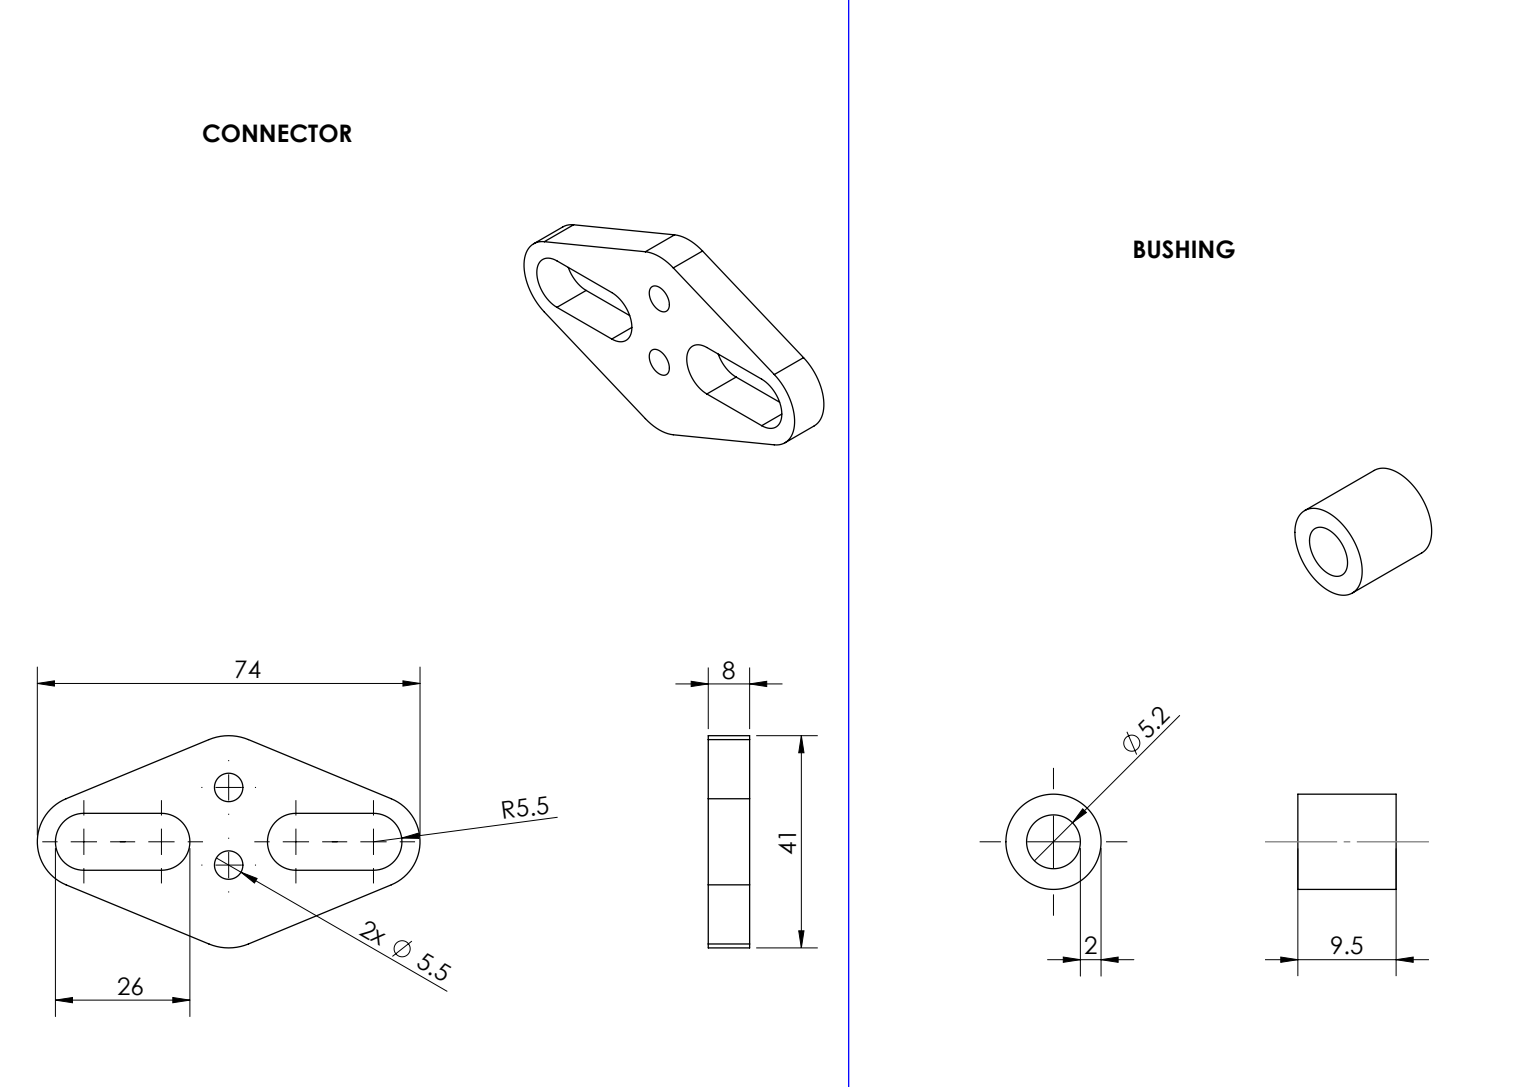
ISO-10303-21;
HEADER;
FILE_DESCRIPTION (('STEP AP214'),
    '1' );
FILE_NAME ('connector.step',
    '2026-09-24T10:26:00',
    ( '' ),
    ( '' ),
    'SwSTEP 2.0',
    'SolidWorks 2026',
    '' );
FILE_SCHEMA (( 'AUTOMOTIVE_DESIGN' ));
ENDSEC;

DATA;
#4=FACE_OUTER_BOUND ( 'NONE', #1590, .T. ) ;
#5=CARTESIAN_POINT ( 'NONE',  ( -13.00000000000000533, 35.49999999999997158, 8.000000000000007105 ) ) ;
#22=CARTESIAN_POINT ( 'NONE',  ( 0.000000000000000000, 25.49999999999996803, 8.000000000000007105 ) ) ;
#36=VERTEX_POINT ( 'NONE', #7746 ) ;
#80=CARTESIAN_POINT ( 'NONE',  ( 2.750000000000003997, 40.49999999999999289, 8.000000000000007105 ) ) ;
#107=EDGE_CURVE ( 'NONE', #8048, #4572, #11469, .T. ) ;
#109=EDGE_CURVE ( 'NONE', #144, #5025, #8095, .T. ) ;
#144=VERTEX_POINT ( 'NONE', #80 ) ;
#167=CARTESIAN_POINT ( 'NONE',  ( 0.000000000000000000, 0.000000000000000000, 0.000000000000000000 ) ) ;
#246=AXIS2_PLACEMENT_3D ( 'NONE', #2195, #9875, #11107 ) ;
#284=VECTOR ( 'NONE', #9089, 1000.000000000000000 ) ;
#288=VECTOR ( 'NONE', #14234, 1000.000000000000000 ) ;
#291=ORIENTED_EDGE ( 'NONE', *, *, #5105, .F. ) ;
#312=EDGE_CURVE ( 'NONE', #10181, #36, #9348, .T. ) ;
#320=ORIENTED_EDGE ( 'NONE', *, *, #6806, .T. ) ;
#341=CARTESIAN_POINT ( 'NONE',  ( 7.500000000000029310, 29.99999999999999289, 0.000000000000000000 ) ) ;
#359=EDGE_LOOP ( 'NONE', ( #6846, #13028, #8516, #4534 ) ) ;
#381=EDGE_CURVE ( 'NONE', #10071, #10068, #6343, .T. ) ;
#397=DIRECTION ( 'NONE',  ( 0.000000000000000000, 0.000000000000000000, -1.000000000000000000 ) ) ;
#405=DIRECTION ( 'NONE',  ( -1.000000000000000000, 0.000000000000000000, 0.000000000000000000 ) ) ;
#413=DIRECTION ( 'NONE',  ( 0.000000000000000000, 0.000000000000000000, 1.000000000000000000 ) ) ;
#414=CARTESIAN_POINT ( 'NONE',  ( -18.12748877629581656, 43.82334295289051340, 8.000000000000007105 ) ) ;
#427=DIRECTION ( 'NONE',  ( 1.000000000000000000, -2.312964634635743450E-16, -0.000000000000000000 ) ) ;
#438=LINE ( 'NONE', #13839, #5839 ) ;
#445=CARTESIAN_POINT ( 'NONE',  ( 28.00000000000000355, 24.50000000000001421, 8.000000000000007105 ) ) ;
#464=AXIS2_PLACEMENT_3D ( 'NONE', #1456, #12793, #10384 ) ;
#503=AXIS2_PLACEMENT_3D ( 'NONE', #5425, #10035, #883 ) ;
#507=CIRCLE ( 'NONE', #2371, 2.750000000000003997 ) ;
#525=CIRCLE ( 'NONE', #4047, 2.749999999999997780 ) ;
#551=ORIENTED_EDGE ( 'NONE', *, *, #3076, .F. ) ;
#572=ORIENTED_EDGE ( 'NONE', *, *, #5224, .F. ) ;
#600=FACE_BOUND ( 'NONE', #2682, .T. ) ;
#610=CARTESIAN_POINT ( 'NONE',  ( 28.00000000000000355, 29.99999999999999645, 8.000000000000007105 ) ) ;
#616=DIRECTION ( 'NONE',  ( -0.3822382184081045131, -0.9240638205168505426, 0.000000000000000000 ) ) ;
#620=EDGE_CURVE ( 'NONE', #11306, #10601, #10148, .T. ) ;
#628=LINE ( 'NONE', #5290, #3064 ) ;
#633=DIRECTION ( 'NONE',  ( 1.000000000000000000, 2.312964634635743943E-16, 0.000000000000000000 ) ) ;
#683=ORIENTED_EDGE ( 'NONE', *, *, #8121, .T. ) ;
#690=CARTESIAN_POINT ( 'NONE',  ( 0.000000000000000000, 40.49999999999999289, 8.000000000000007105 ) ) ;
#697=CARTESIAN_POINT ( 'NONE',  ( -1.734723475976807094E-14, 35.49999999999996447, 8.000000000000007105 ) ) ;
#699=CARTESIAN_POINT ( 'NONE',  ( -28.00000000000000355, 24.50000000000001421, 0.000000000000000000 ) ) ;
#717=DIRECTION ( 'NONE',  ( 0.000000000000000000, 0.000000000000000000, 1.000000000000000000 ) ) ;
#734=AXIS2_PLACEMENT_3D ( 'NONE', #1571, #11524, #13887 ) ;
#780=VERTEX_POINT ( 'NONE', #341 ) ;
#781=ORIENTED_EDGE ( 'NONE', *, *, #5427, .F. ) ;
#791=ORIENTED_EDGE ( 'NONE', *, *, #5224, .T. ) ;
#817=FACE_OUTER_BOUND ( 'NONE', #5758, .T. ) ;
#845=ORIENTED_EDGE ( 'NONE', *, *, #10025, .T. ) ;
#857=DIRECTION ( 'NONE',  ( -0.9240638205168504316, -0.3822382184081046796, 0.000000000000000000 ) ) ;
#880=AXIS2_PLACEMENT_3D ( 'NONE', #8213, #12758, #633 ) ;
#883=DIRECTION ( 'NONE',  ( 1.000000000000000000, 0.000000000000000000, 0.000000000000000000 ) ) ;
#894=LINE ( 'NONE', #5363, #5186 ) ;
#904=VERTEX_POINT ( 'NONE', #6329 ) ;
#912=ADVANCED_FACE ( 'NONE', ( #10802 ), #5239, .T. ) ;
#915=VECTOR ( 'NONE', #4396, 1000.000000000000000 ) ;
#918=DIRECTION ( 'NONE',  ( -0.9240638205168505426, 0.3822382184081045131, 0.000000000000000000 ) ) ;
#937=VERTEX_POINT ( 'NONE', #8951 ) ;
#967=EDGE_CURVE ( 'NONE', #12483, #10071, #11085, .T. ) ;
#974=VERTEX_POINT ( 'NONE', #5712 ) ;
#983=LINE ( 'NONE', #4375, #284 ) ;
#1008=LINE ( 'NONE', #8975, #12593 ) ;
#1020=ADVANCED_FACE ( 'NONE', ( #12260 ), #3623, .T. ) ;
#1027=PRESENTATION_STYLE_ASSIGNMENT (( #3166 ) ) ;
#1039=CARTESIAN_POINT ( 'NONE',  ( -28.00000000000000355, 24.50000000000001421, 8.000000000000007105 ) ) ;
#1069=CYLINDRICAL_SURFACE ( 'NONE', #14439, 5.499999999999980460 ) ;
#1098=LINE ( 'NONE', #5, #8563 ) ;
#1105=CARTESIAN_POINT ( 'NONE',  ( -13.00000000000000533, 29.99999999999999289, 8.000000000000007105 ) ) ;
#1144=DIRECTION ( 'NONE',  ( -1.000000000000000000, 0.000000000000000000, 0.000000000000000000 ) ) ;
#1145=ORIENTED_EDGE ( 'NONE', *, *, #1919, .T. ) ;
#1151=DIRECTION ( 'NONE',  ( 1.000000000000000000, 0.000000000000000000, 0.000000000000000000 ) ) ;
#1155=CARTESIAN_POINT ( 'NONE',  ( -3.822382184081044798, 10.25936179483149324, 8.000000000000007105 ) ) ;
#1205=CARTESIAN_POINT ( 'NONE',  ( 2.750000000000003997, 40.49999999999999289, 0.000000000000000000 ) ) ;
#1262=( NAMED_UNIT ( * ) SI_UNIT ( $, .STERADIAN. ) SOLID_ANGLE_UNIT ( ) );
#1279=DIRECTION ( 'NONE',  ( 0.000000000000000000, 0.000000000000000000, -1.000000000000000000 ) ) ;
#1339=CARTESIAN_POINT ( 'NONE',  ( 6.938893903907228378E-15, 24.50000000000002132, 8.000000000000007105 ) ) ;
#1370=ORIENTED_EDGE ( 'NONE', *, *, #11562, .T. ) ;
#1384=STYLED_ITEM ( 'NONE', ( #1027 ), #1904 ) ;
#1386=EDGE_LOOP ( 'NONE', ( #10991, #9939, #6561, #8171 ) ) ;
#1392=( NAMED_UNIT ( * ) PLANE_ANGLE_UNIT ( ) SI_UNIT ( $, .RADIAN. ) );
#1415=EDGE_CURVE ( 'NONE', #10068, #5462, #7017, .T. ) ;
#1438=LINE ( 'NONE', #7875, #11643 ) ;
#1440=CIRCLE ( 'NONE', #3797, 5.499999999999975131 ) ;
#1456=CARTESIAN_POINT ( 'NONE',  ( -28.00000000000000355, 29.99999999999999645, 8.000000000000007105 ) ) ;
#1461=CARTESIAN_POINT ( 'NONE',  ( 13.00000000000000533, 35.49999999999997158, 0.000000000000000000 ) ) ;
#1463=( GEOMETRIC_REPRESENTATION_CONTEXT ( 3 ) GLOBAL_UNCERTAINTY_ASSIGNED_CONTEXT ( ( #12594 ) ) GLOBAL_UNIT_ASSIGNED_CONTEXT ( ( #1937, #9751, #3116 ) ) REPRESENTATION_CONTEXT ( 'NONE', 'WORKASPACE' ) );
#1500=EDGE_CURVE ( 'NONE', #144, #904, #9130, .T. ) ;
#1522=LINE ( 'NONE', #10104, #2529 ) ;
#1537=EDGE_LOOP ( 'NONE', ( #12834, #4232, #7012, #1145 ) ) ;
#1571=CARTESIAN_POINT ( 'NONE',  ( 28.00000000000000355, 29.99999999999999645, 0.000000000000000000 ) ) ;
#1589=CIRCLE ( 'NONE', #11877, 5.499999999999980460 ) ;
#1590=EDGE_LOOP ( 'NONE', ( #13097, #7525, #7860, #7717 ) ) ;
#1593=EDGE_CURVE ( 'NONE', #5280, #11750, #9299, .T. ) ;
#1607=VECTOR ( 'NONE', #8017, 1000.000000000000000 ) ;
#1629=ADVANCED_FACE ( 'NONE', ( #6815 ), #12659, .F. ) ;
#1635=DIRECTION ( 'NONE',  ( -0.9240638205168504316, -0.3822382184081046796, 0.000000000000000000 ) ) ;
#1657=DIRECTION ( 'NONE',  ( 1.000000000000000000, 0.000000000000000000, 0.000000000000000000 ) ) ;
#1674=EDGE_LOOP ( 'NONE', ( #6926, #2420, #5165, #9689 ) ) ;
#1718=EDGE_LOOP ( 'NONE', ( #3786, #2990 ) ) ;
#1720=DIRECTION ( 'NONE',  ( 0.000000000000000000, 0.000000000000000000, 1.000000000000000000 ) ) ;
#1734=ORIENTED_EDGE ( 'NONE', *, *, #1758, .F. ) ;
#1744=CARTESIAN_POINT ( 'NONE',  ( -13.00000000000000533, 35.49999999999997158, 0.000000000000000000 ) ) ;
#1754=ORIENTED_EDGE ( 'NONE', *, *, #3468, .T. ) ;
#1758=EDGE_CURVE ( 'NONE', #10181, #11306, #2144, .T. ) ;
#1788=VERTEX_POINT ( 'NONE', #12898 ) ;
#1802=ORIENTED_EDGE ( 'NONE', *, *, #10042, .T. ) ;
#1808=CARTESIAN_POINT ( 'NONE',  ( 13.00000000000000533, 29.99999999999999289, 0.000000000000000000 ) ) ;
#1828=FACE_OUTER_BOUND ( 'NONE', #10687, .T. ) ;
#1840=VERTEX_POINT ( 'NONE', #14283 ) ;
#1860=FILL_AREA_STYLE_COLOUR ( '', #12668 ) ;
#1865=VERTEX_POINT ( 'NONE', #8711 ) ;
#1880=VECTOR ( 'NONE', #857, 1000.000000000000114 ) ;
#1898=DIRECTION ( 'NONE',  ( -1.000000000000000000, 0.000000000000000000, 0.000000000000000000 ) ) ;
#1904=MANIFOLD_SOLID_BREP ( 'Boss-Extrude1', #11798 ) ;
#1919=EDGE_CURVE ( 'NONE', #1840, #11047, #9738, .T. ) ;
#1920=CIRCLE ( 'NONE', #8926, 9.000000000000005329 ) ;
#1937=( LENGTH_UNIT ( ) NAMED_UNIT ( * ) SI_UNIT ( .MILLI., .METRE. ) );
#1951=DIRECTION ( 'NONE',  ( 0.000000000000000000, 0.000000000000000000, -1.000000000000000000 ) ) ;
#2011=DIRECTION ( 'NONE',  ( 0.000000000000000000, 0.000000000000000000, -1.000000000000000000 ) ) ;
#2038=AXIS2_PLACEMENT_3D ( 'NONE', #3992, #397, #8135 ) ;
#2042=CYLINDRICAL_SURFACE ( 'NONE', #4497, 5.499999999999984013 ) ;
#2062=VECTOR ( 'NONE', #11153, 1000.000000000000000 ) ;
#2101=DIRECTION ( 'NONE',  ( 0.000000000000000000, 0.000000000000000000, -1.000000000000000000 ) ) ;
#2138=ORIENTED_EDGE ( 'NONE', *, *, #2659, .F. ) ;
#2139=EDGE_CURVE ( 'NONE', #5220, #1840, #12145, .T. ) ;
#2144=CIRCLE ( 'NONE', #4024, 9.000000000000001776 ) ;
#2195=CARTESIAN_POINT ( 'NONE',  ( 0.000000000000000000, 40.49999999999999289, 0.000000000000000000 ) ) ;
#2208=( NAMED_UNIT ( * ) PLANE_ANGLE_UNIT ( ) SI_UNIT ( $, .RADIAN. ) );
#2218=DIRECTION ( 'NONE',  ( 1.000000000000000000, 0.000000000000000000, 0.000000000000000000 ) ) ;
#2236=DIRECTION ( 'NONE',  ( 1.000000000000000000, -2.312964634635743450E-16, -0.000000000000000000 ) ) ;
#2249=CARTESIAN_POINT ( 'NONE',  ( 3.065261730689029740, 7.410293710401357536, 8.000000000000007105 ) ) ;
#2265=ORIENTED_EDGE ( 'NONE', *, *, #3430, .T. ) ;
#2267=VERTEX_POINT ( 'NONE', #14409 ) ;
#2289=CIRCLE ( 'NONE', #8370, 5.499999999999976907 ) ;
#2321=LINE ( 'NONE', #5533, #13804 ) ;
#2334=CARTESIAN_POINT ( 'NONE',  ( 2.750000000000003997, 40.49999999999999289, 8.000000000000007105 ) ) ;
#2360=DIRECTION ( 'NONE',  ( -0.3822382184081050127, -0.9240638205168504316, 0.000000000000000000 ) ) ;
#2361=SURFACE_STYLE_USAGE ( .BOTH. , #7982 ) ;
#2371=AXIS2_PLACEMENT_3D ( 'NONE', #11928, #6421, #14269 ) ;
#2400=LINE ( 'NONE', #3434, #11888 ) ;
#2420=ORIENTED_EDGE ( 'NONE', *, *, #8347, .T. ) ;
#2442=DIRECTION ( 'NONE',  ( -1.000000000000000000, 0.000000000000000000, 0.000000000000000000 ) ) ;
#2462=ORIENTED_EDGE ( 'NONE', *, *, #5881, .T. ) ;
#2474=LINE ( 'NONE', #6923, #10329 ) ;
#2493=ORIENTED_EDGE ( 'NONE', *, *, #10301, .F. ) ;
#2496=DIRECTION ( 'NONE',  ( 0.000000000000000000, 0.000000000000000000, -1.000000000000000000 ) ) ;
#2500=AXIS2_PLACEMENT_3D ( 'NONE', #13365, #11609, #5811 ) ;
#2529=VECTOR ( 'NONE', #427, 1000.000000000000000 ) ;
#2566=( GEOMETRIC_REPRESENTATION_CONTEXT ( 3 ) GLOBAL_UNCERTAINTY_ASSIGNED_CONTEXT ( ( #6305 ) ) GLOBAL_UNIT_ASSIGNED_CONTEXT ( ( #10838, #2208, #14357 ) ) REPRESENTATION_CONTEXT ( 'NONE', 'WORKASPACE' ) );
#2587=AXIS2_PLACEMENT_3D ( 'NONE', #7667, #4199, #14427 ) ;
#2592=DIRECTION ( 'NONE',  ( 1.000000000000000000, 0.000000000000000000, 0.000000000000000000 ) ) ;
#2659=EDGE_CURVE ( 'NONE', #12223, #11750, #9069, .T. ) ;
#2672=DIRECTION ( 'NONE',  ( -1.000000000000000000, 0.000000000000000000, 0.000000000000000000 ) ) ;
#2677=CARTESIAN_POINT ( 'NONE',  ( 7.500000000000029310, 29.99999999999999289, 8.000000000000007105 ) ) ;
#2682=EDGE_LOOP ( 'NONE', ( #6005, #6143, #572, #4410, #10204 ) ) ;
#2690=ORIENTED_EDGE ( 'NONE', *, *, #11605, .T. ) ;
#2714=CARTESIAN_POINT ( 'NONE',  ( -3.822382184081044798, 10.25936179483149324, 0.000000000000000000 ) ) ;
#2721=ADVANCED_FACE ( 'NONE', ( #9165 ), #11227, .T. ) ;
#2767=DIRECTION ( 'NONE',  ( 0.000000000000000000, 0.000000000000000000, -1.000000000000000000 ) ) ;
#2778=AXIS2_PLACEMENT_3D ( 'NONE', #3914, #4929, #9316 ) ;
#2799=EDGE_CURVE ( 'NONE', #12483, #8354, #12334, .T. ) ;
#2801=DIRECTION ( 'NONE',  ( 0.000000000000000000, 0.000000000000000000, 1.000000000000000000 ) ) ;
#2811=CARTESIAN_POINT ( 'NONE',  ( 28.00000000000000355, 29.99999999999999645, 0.000000000000000000 ) ) ;
#2835=EDGE_LOOP ( 'NONE', ( #7365, #10921, #3475, #8407 ) ) ;
#2865=CARTESIAN_POINT ( 'NONE',  ( 18.12748877629582367, 43.82334295289049919, 8.000000000000007105 ) ) ;
#2868=SHAPE_DEFINITION_REPRESENTATION ( #11381, #7856 ) ;
#2871=ORIENTED_EDGE ( 'NONE', *, *, #10301, .T. ) ;
#2876=ADVANCED_FACE ( 'NONE', ( #8284 ), #10414, .F. ) ;
#2905=ORIENTED_EDGE ( 'NONE', *, *, #9218, .F. ) ;
#2921=ORIENTED_EDGE ( 'NONE', *, *, #9960, .T. ) ;
#2945=FACE_BOUND ( 'NONE', #7169, .T. ) ;
#2956=ADVANCED_FACE ( 'NONE', ( #6170 ), #14023, .F. ) ;
#2971=LINE ( 'NONE', #6388, #288 ) ;
#2990=ORIENTED_EDGE ( 'NONE', *, *, #1500, .F. ) ;
#3024=AXIS2_PLACEMENT_3D ( 'NONE', #1105, #8786, #8854 ) ;
#3035=CARTESIAN_POINT ( 'NONE',  ( 13.00000000000000533, 29.99999999999999289, 0.000000000000000000 ) ) ;
#3055=CARTESIAN_POINT ( 'NONE',  ( 3.065261730689029740, 7.410293710401357536, 0.000000000000000000 ) ) ;
#3063=CARTESIAN_POINT ( 'NONE',  ( 0.000000000000000000, 25.49999999999996803, 0.000000000000000000 ) ) ;
#3064=VECTOR ( 'NONE', #10854, 1000.000000000000000 ) ;
#3076=EDGE_CURVE ( 'NONE', #1865, #9330, #1098, .T. ) ;
#3103=AXIS2_PLACEMENT_3D ( 'NONE', #14152, #616, #4062 ) ;
#3116=( NAMED_UNIT ( * ) SI_UNIT ( $, .STERADIAN. ) SOLID_ANGLE_UNIT ( ) );
#3160=DIRECTION ( 'NONE',  ( 1.000000000000000000, 0.000000000000000000, 0.000000000000000000 ) ) ;
#3166=SURFACE_STYLE_USAGE ( .BOTH. , #3232 ) ;
#3171=ADVANCED_FACE ( 'NONE', ( #5288 ), #5007, .T. ) ;
#3205=DIRECTION ( 'NONE',  ( -0.9240638205168504316, -0.3822382184081047352, 0.000000000000000000 ) ) ;
#3222=VECTOR ( 'NONE', #5160, 1000.000000000000000 ) ;
#3225=VERTEX_POINT ( 'NONE', #9607 ) ;
#3232=SURFACE_SIDE_STYLE ('',( #11050 ) ) ;
#3254=LINE ( 'NONE', #9693, #13621 ) ;
#3276=AXIS2_PLACEMENT_3D ( 'NONE', #2865, #2360, #3959 ) ;
#3292=CARTESIAN_POINT ( 'NONE',  ( -13.00000000000000533, 29.99999999999999289, 0.000000000000000000 ) ) ;
#3296=EDGE_LOOP ( 'NONE', ( #5557, #14094 ) ) ;
#3315=ORIENTED_EDGE ( 'NONE', *, *, #1758, .T. ) ;
#3322=LINE ( 'NONE', #1039, #12219 ) ;
#3369=FACE_OUTER_BOUND ( 'NONE', #6945, .T. ) ;
#3370=EDGE_CURVE ( 'NONE', #10504, #11904, #6227, .T. ) ;
#3430=EDGE_CURVE ( 'NONE', #3225, #9041, #1920, .T. ) ;
#3434=CARTESIAN_POINT ( 'NONE',  ( -1.734723475976807094E-14, 35.49999999999996447, 0.000000000000000000 ) ) ;
#3468=EDGE_CURVE ( 'NONE', #7396, #1865, #3793, .T. ) ;
#3475=ORIENTED_EDGE ( 'NONE', *, *, #620, .F. ) ;
#3480=ORIENTED_EDGE ( 'NONE', *, *, #7933, .F. ) ;
#3488=DIRECTION ( 'NONE',  ( -1.000000000000000000, 2.312964634635743943E-16, 0.000000000000000000 ) ) ;
#3527=EDGE_LOOP ( 'NONE', ( #7676, #8823, #7369, #8131 ) ) ;
#3557=DIRECTION ( 'NONE',  ( 0.000000000000000000, 0.000000000000000000, -1.000000000000000000 ) ) ;
#3571=EDGE_LOOP ( 'NONE', ( #14354, #5002 ) ) ;
#3623=CYLINDRICAL_SURFACE ( 'NONE', #9197, 9.000000000000001776 ) ;
#3629=APPLICATION_CONTEXT ( 'automotive_design' ) ;
#3671=AXIS2_PLACEMENT_3D ( 'NONE', #14442, #5568, #10111 ) ;
#3681=VECTOR ( 'NONE', #918, 1000.000000000000000 ) ;
#3685=EDGE_CURVE ( 'NONE', #6397, #10504, #983, .T. ) ;
#3693=CARTESIAN_POINT ( 'NONE',  ( -28.00000000000000355, 29.99999999999999645, 8.000000000000007105 ) ) ;
#3696=CARTESIAN_POINT ( 'NONE',  ( -28.00000000000000355, 29.99999999999999645, 0.000000000000000000 ) ) ;
#3731=FACE_BOUND ( 'NONE', #1718, .T. ) ;
#3785=ORIENTED_EDGE ( 'NONE', *, *, #9218, .T. ) ;
#3786=ORIENTED_EDGE ( 'NONE', *, *, #11283, .F. ) ;
#3793=CIRCLE ( 'NONE', #13617, 5.499999999999975131 ) ;
#3797=AXIS2_PLACEMENT_3D ( 'NONE', #3292, #6708, #4399 ) ;
#3811=FACE_BOUND ( 'NONE', #12655, .T. ) ;
#3820=STYLED_ITEM ( 'NONE', ( #6669 ), #13112 ) ;
#3851=PLANE ( 'NONE',  #880 ) ;
#3861=ORIENTED_EDGE ( 'NONE', *, *, #8889, .T. ) ;
#3879=ADVANCED_FACE ( 'NONE', ( #6895 ), #12916, .F. ) ;
#3880=ORIENTED_EDGE ( 'NONE', *, *, #1415, .F. ) ;
#3914=CARTESIAN_POINT ( 'NONE',  ( 13.00000000000000533, 29.99999999999999289, 8.000000000000007105 ) ) ;
#3945=DIRECTION ( 'NONE',  ( 1.000000000000000000, 4.625929269271485914E-16, 0.000000000000000000 ) ) ;
#3955=CARTESIAN_POINT ( 'NONE',  ( 28.00000000000000355, 35.49999999999997868, 0.000000000000000000 ) ) ;
#3959=DIRECTION ( 'NONE',  ( 0.9240638205168503205, -0.3822382184081049572, -0.000000000000000000 ) ) ;
#3963=DIRECTION ( 'NONE',  ( 0.000000000000000000, 0.000000000000000000, 1.000000000000000000 ) ) ;
#3986=CARTESIAN_POINT ( 'NONE',  ( -28.00000000000000355, 29.99999999999999645, 8.000000000000007105 ) ) ;
#3987=EDGE_LOOP ( 'NONE', ( #11996, #8439, #12869, #2493 ) ) ;
#3992=CARTESIAN_POINT ( 'NONE',  ( -28.00000000000000355, 29.99999999999999645, 8.000000000000007105 ) ) ;
#3994=ORIENTED_EDGE ( 'NONE', *, *, #1415, .T. ) ;
#4015=CIRCLE ( 'NONE', #11708, 2.749999999999997780 ) ;
#4024=AXIS2_PLACEMENT_3D ( 'NONE', #610, #2801, #7241 ) ;
#4040=CARTESIAN_POINT ( 'NONE',  ( 31.44014396567294867, 21.68342561534834090, 8.000000000000007105 ) ) ;
#4047=AXIS2_PLACEMENT_3D ( 'NONE', #22, #10114, #7082 ) ;
#4062=DIRECTION ( 'NONE',  ( 0.9240638205168505426, -0.3822382184081045131, -0.000000000000000000 ) ) ;
#4120=PLANE ( 'NONE',  #4507 ) ;
#4121=CARTESIAN_POINT ( 'NONE',  ( -28.00000000000000355, 29.99999999999999645, 8.000000000000007105 ) ) ;
#4156=ORIENTED_EDGE ( 'NONE', *, *, #11847, .T. ) ;
#4188=ORIENTED_EDGE ( 'NONE', *, *, #6813, .F. ) ;
#4199=DIRECTION ( 'NONE',  ( 0.000000000000000000, 0.000000000000000000, -1.000000000000000000 ) ) ;
#4220=EDGE_CURVE ( 'NONE', #10601, #12223, #11489, .T. ) ;
#4232=ORIENTED_EDGE ( 'NONE', *, *, #5600, .F. ) ;
#4233=DIRECTION ( 'NONE',  ( 1.000000000000000000, 0.000000000000000000, 0.000000000000000000 ) ) ;
#4275=CYLINDRICAL_SURFACE ( 'NONE', #2587, 2.749999999999997780 ) ;
#4296=ORIENTED_EDGE ( 'NONE', *, *, #8889, .F. ) ;
#4326=LINE ( 'NONE', #7645, #7461 ) ;
#4375=CARTESIAN_POINT ( 'NONE',  ( -33.49999999999998579, 29.99999999999999645, 8.000000000000007105 ) ) ;
#4389=ORIENTED_EDGE ( 'NONE', *, *, #5881, .F. ) ;
#4396=DIRECTION ( 'NONE',  ( -1.000000000000000000, 4.625929269271485914E-16, 0.000000000000000000 ) ) ;
#4399=DIRECTION ( 'NONE',  ( 1.000000000000000000, 0.000000000000000000, 0.000000000000000000 ) ) ;
#4406=ORIENTED_EDGE ( 'NONE', *, *, #5896, .F. ) ;
#4410=ORIENTED_EDGE ( 'NONE', *, *, #10256, .T. ) ;
#4414=FILL_AREA_STYLE_COLOUR ( '', #8162 ) ;
#4497=AXIS2_PLACEMENT_3D ( 'NONE', #4121, #8558, #13039 ) ;
#4507=AXIS2_PLACEMENT_3D ( 'NONE', #8324, #3963, #7151 ) ;
#4508=CARTESIAN_POINT ( 'NONE',  ( 28.00000000000000355, 24.50000000000001421, 0.000000000000000000 ) ) ;
#4534=ORIENTED_EDGE ( 'NONE', *, *, #4220, .T. ) ;
#4537=DIRECTION ( 'NONE',  ( -0.9240638205168503205, 0.3822382184081049017, 0.000000000000000000 ) ) ;
#4572=VERTEX_POINT ( 'NONE', #7821 ) ;
#4604=LINE ( 'NONE', #7808, #915 ) ;
#4641=FACE_OUTER_BOUND ( 'NONE', #12693, .T. ) ;
#4692=ORIENTED_EDGE ( 'NONE', *, *, #13091, .F. ) ;
#4693=EDGE_CURVE ( 'NONE', #11306, #2267, #438, .T. ) ;
#4708=VECTOR ( 'NONE', #2496, 1000.000000000000000 ) ;
#4725=DIRECTION ( 'NONE',  ( 0.000000000000000000, 0.000000000000000000, -1.000000000000000000 ) ) ;
#4738=CIRCLE ( 'NONE', #13393, 9.999999999999996447 ) ;
#4743=DIRECTION ( 'NONE',  ( 0.000000000000000000, 0.000000000000000000, -1.000000000000000000 ) ) ;
#4752=ORIENTED_EDGE ( 'NONE', *, *, #1593, .T. ) ;
#4771=DIRECTION ( 'NONE',  ( 0.000000000000000000, 0.000000000000000000, -1.000000000000000000 ) ) ;
#4772=CARTESIAN_POINT ( 'NONE',  ( 0.000000000000000000, 40.49999999999999289, 8.000000000000007105 ) ) ;
#4779=ORIENTED_EDGE ( 'NONE', *, *, #6806, .F. ) ;
#4791=ORIENTED_EDGE ( 'NONE', *, *, #6813, .T. ) ;
#4798=EDGE_LOOP ( 'NONE', ( #1802, #12381, #9453, #10952 ) ) ;
#4800=ORIENTED_EDGE ( 'NONE', *, *, #381, .F. ) ;
#4816=DIRECTION ( 'NONE',  ( 0.000000000000000000, 0.000000000000000000, -1.000000000000000000 ) ) ;
#4834=EDGE_CURVE ( 'NONE', #937, #4572, #4015, .T. ) ;
#4843=EDGE_CURVE ( 'NONE', #904, #8755, #6404, .T. ) ;
#4875=DIRECTION ( 'NONE',  ( 0.3822382184081047352, -0.9240638205168505426, -0.000000000000000000 ) ) ;
#4927=AXIS2_PLACEMENT_3D ( 'NONE', #14166, #8365, #6316 ) ;
#4929=DIRECTION ( 'NONE',  ( 0.000000000000000000, 0.000000000000000000, -1.000000000000000000 ) ) ;
#4931=DIRECTION ( 'NONE',  ( 1.000000000000000000, 0.000000000000000000, 0.000000000000000000 ) ) ;
#4947=DIRECTION ( 'NONE',  ( 1.000000000000000000, 0.000000000000000000, 0.000000000000000000 ) ) ;
#4955=AXIS2_PLACEMENT_3D ( 'NONE', #13724, #9243, #2592 ) ;
#4990=PRODUCT_DEFINITION ( 'UNKNOWN', '', #9904, #13349 ) ;
#4996=VERTEX_POINT ( 'NONE', #6754 ) ;
#5002=ORIENTED_EDGE ( 'NONE', *, *, #9870, .F. ) ;
#5007=CYLINDRICAL_SURFACE ( 'NONE', #6448, 9.000000000000001776 ) ;
#5024=CARTESIAN_POINT ( 'NONE',  ( -13.00000000000000533, 29.99999999999999289, 8.000000000000007105 ) ) ;
#5025=VERTEX_POINT ( 'NONE', #1205 ) ;
#5041=LINE ( 'NONE', #6346, #6303 ) ;
#5071=ORIENTED_EDGE ( 'NONE', *, *, #14458, .T. ) ;
#5105=EDGE_CURVE ( 'NONE', #6397, #9797, #1589, .T. ) ;
#5110=DIRECTION ( 'NONE',  ( 0.000000000000000000, 0.000000000000000000, -1.000000000000000000 ) ) ;
#5151=DIRECTION ( 'NONE',  ( -1.000000000000000000, -4.625929269271486900E-16, 0.000000000000000000 ) ) ;
#5152=ORIENTED_EDGE ( 'NONE', *, *, #7917, .T. ) ;
#5153=AXIS2_PLACEMENT_3D ( 'NONE', #12494, #12427, #9042 ) ;
#5160=DIRECTION ( 'NONE',  ( -0.9240638205168505426, 0.3822382184081045131, 0.000000000000000000 ) ) ;
#5165=ORIENTED_EDGE ( 'NONE', *, *, #2799, .T. ) ;
#5186=VECTOR ( 'NONE', #13070, 1000.000000000000000 ) ;
#5220=VERTEX_POINT ( 'NONE', #10641 ) ;
#5224=EDGE_CURVE ( 'NONE', #974, #11904, #628, .T. ) ;
#5239=CYLINDRICAL_SURFACE ( 'NONE', #13893, 10.00000000000000355 ) ;
#5280=VERTEX_POINT ( 'NONE', #10605 ) ;
#5288=FACE_OUTER_BOUND ( 'NONE', #13955, .T. ) ;
#5290=CARTESIAN_POINT ( 'NONE',  ( -6.938893903907228378E-15, 24.50000000000002132, 0.000000000000000000 ) ) ;
#5293=ORIENTED_EDGE ( 'NONE', *, *, #5636, .F. ) ;
#5308=DIRECTION ( 'NONE',  ( 0.000000000000000000, 0.000000000000000000, 1.000000000000000000 ) ) ;
#5326=CYLINDRICAL_SURFACE ( 'NONE', #6984, 9.999999999999996447 ) ;
#5347=ADVANCED_FACE ( 'NONE', ( #3731, #12505, #7002, #3811, #12639 ), #5900, .T. ) ;
#5363=CARTESIAN_POINT ( 'NONE',  ( -28.00000000000000355, 35.49999999999997868, 8.000000000000007105 ) ) ;
#5425=CARTESIAN_POINT ( 'NONE',  ( 0.000000000000000000, 40.49999999999999289, 8.000000000000007105 ) ) ;
#5427=EDGE_CURVE ( 'NONE', #7396, #9797, #5041, .T. ) ;
#5441=DIRECTION ( 'NONE',  ( 1.000000000000000000, 0.000000000000000000, 0.000000000000000000 ) ) ;
#5462=VERTEX_POINT ( 'NONE', #3955 ) ;
#5481=EDGE_CURVE ( 'NONE', #11750, #3225, #6479, .T. ) ;
#5512=ORIENTED_EDGE ( 'NONE', *, *, #967, .F. ) ;
#5533=CARTESIAN_POINT ( 'NONE',  ( -3.822382184081044798, 10.25936179483149324, 8.000000000000007105 ) ) ;
#5557=ORIENTED_EDGE ( 'NONE', *, *, #13465, .T. ) ;
#5568=DIRECTION ( 'NONE',  ( 0.000000000000000000, 0.000000000000000000, 1.000000000000000000 ) ) ;
#5600=EDGE_CURVE ( 'NONE', #11470, #11163, #2321, .T. ) ;
#5615=DIRECTION ( 'NONE',  ( 0.000000000000000000, 0.000000000000000000, -1.000000000000000000 ) ) ;
#5631=CARTESIAN_POINT ( 'NONE',  ( -2.749999999999997780, 25.49999999999996803, 8.000000000000007105 ) ) ;
#5636=EDGE_CURVE ( 'NONE', #2267, #12223, #4326, .T. ) ;
#5712=CARTESIAN_POINT ( 'NONE',  ( -13.00000000000000533, 24.50000000000001421, 0.000000000000000000 ) ) ;
#5716=DIRECTION ( 'NONE',  ( 2.312964634635743943E-16, 1.000000000000000000, 0.000000000000000000 ) ) ;
#5749=CARTESIAN_POINT ( 'NONE',  ( -31.44014396567295577, 21.68342561534834445, 8.000000000000007105 ) ) ;
#5758=EDGE_LOOP ( 'NONE', ( #10144, #11076, #1754, #6948 ) ) ;
#5803=ADVANCED_FACE ( 'NONE', ( #9260 ), #8155, .F. ) ;
#5811=DIRECTION ( 'NONE',  ( 1.000000000000000000, 0.000000000000000000, 0.000000000000000000 ) ) ;
#5839=VECTOR ( 'NONE', #7892, 1000.000000000000000 ) ;
#5869=ORIENTED_EDGE ( 'NONE', *, *, #13068, .T. ) ;
#5881=EDGE_CURVE ( 'NONE', #11189, #780, #8881, .T. ) ;
#5888=LINE ( 'NONE', #13685, #7711 ) ;
#5894=CARTESIAN_POINT ( 'NONE',  ( 13.00000000000000533, 29.99999999999999289, 8.000000000000007105 ) ) ;
#5896=EDGE_CURVE ( 'NONE', #8969, #5220, #8182, .T. ) ;
#5899=ORIENTED_EDGE ( 'NONE', *, *, #9224, .T. ) ;
#5900=PLANE ( 'NONE',  #464 ) ;
#6005=ORIENTED_EDGE ( 'NONE', *, *, #6624, .T. ) ;
#6009=CARTESIAN_POINT ( 'NONE',  ( -28.00000000000000355, 24.50000000000001421, 8.000000000000007105 ) ) ;
#6019=AXIS2_PLACEMENT_3D ( 'NONE', #9392, #12602, #2672 ) ;
#6060=ORIENTED_EDGE ( 'NONE', *, *, #7237, .F. ) ;
#6143=ORIENTED_EDGE ( 'NONE', *, *, #3370, .T. ) ;
#6170=FACE_OUTER_BOUND ( 'NONE', #11038, .T. ) ;
#6173=EDGE_CURVE ( 'NONE', #5280, #8969, #14019, .T. ) ;
#6227=CIRCLE ( 'NONE', #3671, 5.499999999999980460 ) ;
#6242=VECTOR ( 'NONE', #3205, 1000.000000000000000 ) ;
#6294=CIRCLE ( 'NONE', #11666, 5.499999999999980460 ) ;
#6303=VECTOR ( 'NONE', #9721, 1000.000000000000000 ) ;
#6305=UNCERTAINTY_MEASURE_WITH_UNIT (LENGTH_MEASURE( 1.000000000000000082E-05 ), #10838, 'distance_accuracy_value', 'NONE');
#6312=SURFACE_STYLE_FILL_AREA ( #6599 ) ;
#6316=DIRECTION ( 'NONE',  ( -1.000000000000000000, 0.000000000000000000, 0.000000000000000000 ) ) ;
#6329=CARTESIAN_POINT ( 'NONE',  ( -2.750000000000003997, 40.49999999999999289, 8.000000000000007105 ) ) ;
#6343=LINE ( 'NONE', #7726, #13187 ) ;
#6346=CARTESIAN_POINT ( 'NONE',  ( -6.938893903907228378E-15, 24.50000000000002132, 8.000000000000007105 ) ) ;
#6348=CIRCLE ( 'NONE', #4955, 2.749999999999997780 ) ;
#6369=( GEOMETRIC_REPRESENTATION_CONTEXT ( 3 ) GLOBAL_UNCERTAINTY_ASSIGNED_CONTEXT ( ( #10848 ) ) GLOBAL_UNIT_ASSIGNED_CONTEXT ( ( #11208, #1392, #1262 ) ) REPRESENTATION_CONTEXT ( 'NONE', 'WORKASPACE' ) );
#6388=CARTESIAN_POINT ( 'NONE',  ( 1.734723475976807094E-14, 35.49999999999996447, 8.000000000000007105 ) ) ;
#6397=VERTEX_POINT ( 'NONE', #9510 ) ;
#6399=DIRECTION ( 'NONE',  ( -1.000000000000000000, 0.000000000000000000, 0.000000000000000000 ) ) ;
#6404=LINE ( 'NONE', #7144, #7251 ) ;
#6414=ADVANCED_FACE ( 'NONE', ( #8399 ), #10179, .F. ) ;
#6421=DIRECTION ( 'NONE',  ( 0.000000000000000000, 0.000000000000000000, 1.000000000000000000 ) ) ;
#6448=AXIS2_PLACEMENT_3D ( 'NONE', #3986, #8431, #7400 ) ;
#6479=LINE ( 'NONE', #7580, #1880 ) ;
#6484=AXIS2_PLACEMENT_3D ( 'NONE', #3696, #1720, #4931 ) ;
#6524=DIRECTION ( 'NONE',  ( 0.000000000000000000, 0.000000000000000000, 1.000000000000000000 ) ) ;
#6544=ADVANCED_FACE ( 'NONE', ( #1828 ), #5326, .T. ) ;
#6545=DIRECTION ( 'NONE',  ( 0.000000000000000000, 0.000000000000000000, 1.000000000000000000 ) ) ;
#6552=DIRECTION ( 'NONE',  ( 0.000000000000000000, 0.000000000000000000, -1.000000000000000000 ) ) ;
#6556=DIRECTION ( 'NONE',  ( 0.000000000000000000, 0.000000000000000000, -1.000000000000000000 ) ) ;
#6561=ORIENTED_EDGE ( 'NONE', *, *, #967, .T. ) ;
#6588=CARTESIAN_POINT ( 'NONE',  ( 0.000000000000000000, 19.49999999999999645, 0.000000000000000000 ) ) ;
#6589=CARTESIAN_POINT ( 'NONE',  ( 2.749999999999997780, 25.49999999999996803, 8.000000000000007105 ) ) ;
#6599=FILL_AREA_STYLE ('',( #1860 ) ) ;
#6624=EDGE_CURVE ( 'NONE', #1788, #10504, #6294, .T. ) ;
#6631=EDGE_CURVE ( 'NONE', #14193, #937, #1008, .T. ) ;
#6669=PRESENTATION_STYLE_ASSIGNMENT (( #2361 ) ) ;
#6684=CARTESIAN_POINT ( 'NONE',  ( 6.938893903907228378E-15, 24.50000000000002132, 8.000000000000007105 ) ) ;
#6693=CARTESIAN_POINT ( 'NONE',  ( -3.065261730689029740, 7.410293710401353984, 0.000000000000000000 ) ) ;
#6695=ORIENTED_EDGE ( 'NONE', *, *, #7933, .T. ) ;
#6708=DIRECTION ( 'NONE',  ( 0.000000000000000000, 0.000000000000000000, 1.000000000000000000 ) ) ;
#6727=ADVANCED_FACE ( 'NONE', ( #3369 ), #7548, .T. ) ;
#6732=DIRECTION ( 'NONE',  ( 0.000000000000000000, 0.000000000000000000, 1.000000000000000000 ) ) ;
#6735=EDGE_CURVE ( 'NONE', #9330, #1788, #4604, .T. ) ;
#6754=CARTESIAN_POINT ( 'NONE',  ( -28.00000000000000355, 35.49999999999997868, 8.000000000000007105 ) ) ;
#6806=EDGE_CURVE ( 'NONE', #5220, #9041, #13896, .T. ) ;
#6813=EDGE_CURVE ( 'NONE', #9740, #5462, #10590, .T. ) ;
#6815=FACE_OUTER_BOUND ( 'NONE', #13835, .T. ) ;
#6846=ORIENTED_EDGE ( 'NONE', *, *, #2659, .T. ) ;
#6853=VECTOR ( 'NONE', #8478, 1000.000000000000000 ) ;
#6866=ORIENTED_EDGE ( 'NONE', *, *, #3370, .F. ) ;
#6877=CARTESIAN_POINT ( 'NONE',  ( -31.44014396567295577, 21.68342561534834445, 0.000000000000000000 ) ) ;
#6895=FACE_OUTER_BOUND ( 'NONE', #3987, .T. ) ;
#6923=CARTESIAN_POINT ( 'NONE',  ( -1.734723475976807094E-14, 35.49999999999996447, 8.000000000000007105 ) ) ;
#6926=ORIENTED_EDGE ( 'NONE', *, *, #11847, .F. ) ;
#6929=VERTEX_POINT ( 'NONE', #8987 ) ;
#6945=EDGE_LOOP ( 'NONE', ( #9380, #9174, #9627, #11572 ) ) ;
#6948=ORIENTED_EDGE ( 'NONE', *, *, #3076, .T. ) ;
#6984=AXIS2_PLACEMENT_3D ( 'NONE', #9582, #5110, #1898 ) ;
#7002=FACE_OUTER_BOUND ( 'NONE', #9276, .T. ) ;
#7012=ORIENTED_EDGE ( 'NONE', *, *, #8323, .T. ) ;
#7017=CIRCLE ( 'NONE', #734, 5.499999999999984013 ) ;
#7082=DIRECTION ( 'NONE',  ( 1.000000000000000000, 0.000000000000000000, 0.000000000000000000 ) ) ;
#7115=CARTESIAN_POINT ( 'NONE',  ( 3.822382184081044798, 10.25936179483148969, 8.000000000000007105 ) ) ;
#7126=VERTEX_POINT ( 'NONE', #2677 ) ;
#7136=CARTESIAN_POINT ( 'NONE',  ( -33.49999999999998579, 29.99999999999999645, 0.000000000000000000 ) ) ;
#7144=CARTESIAN_POINT ( 'NONE',  ( -2.750000000000003997, 40.49999999999999289, 8.000000000000007105 ) ) ;
#7151=DIRECTION ( 'NONE',  ( 1.000000000000000000, 0.000000000000000000, 0.000000000000000000 ) ) ;
#7169=EDGE_LOOP ( 'NONE', ( #6695, #2871 ) ) ;
#7186=CARTESIAN_POINT ( 'NONE',  ( 28.00000000000000355, 35.49999999999997868, 8.000000000000007105 ) ) ;
#7211=VECTOR ( 'NONE', #2767, 1000.000000000000000 ) ;
#7225=CARTESIAN_POINT ( 'NONE',  ( -28.00000000000000355, 29.99999999999999645, 8.000000000000007105 ) ) ;
#7230=FACE_OUTER_BOUND ( 'NONE', #12906, .T. ) ;
#7237=EDGE_CURVE ( 'NONE', #36, #11314, #12687, .T. ) ;
#7241=DIRECTION ( 'NONE',  ( 1.000000000000000000, 0.000000000000000000, 0.000000000000000000 ) ) ;
#7251=VECTOR ( 'NONE', #9922, 1000.000000000000000 ) ;
#7270=CARTESIAN_POINT ( 'NONE',  ( -13.00000000000000533, 24.50000000000001421, 8.000000000000007105 ) ) ;
#7303=ORIENTED_EDGE ( 'NONE', *, *, #5600, .T. ) ;
#7322=AXIS2_PLACEMENT_3D ( 'NONE', #2811, #9157, #13653 ) ;
#7345=VECTOR ( 'NONE', #5615, 1000.000000000000000 ) ;
#7365=ORIENTED_EDGE ( 'NONE', *, *, #5636, .T. ) ;
#7369=ORIENTED_EDGE ( 'NONE', *, *, #6624, .F. ) ;
#7396=VERTEX_POINT ( 'NONE', #7270 ) ;
#7400=DIRECTION ( 'NONE',  ( -1.000000000000000000, 0.000000000000000000, 0.000000000000000000 ) ) ;
#7405=FACE_OUTER_BOUND ( 'NONE', #13889, .T. ) ;
#7407=ORIENTED_EDGE ( 'NONE', *, *, #5481, .T. ) ;
#7421=CARTESIAN_POINT ( 'NONE',  ( -28.00000000000000355, 29.99999999999999645, 8.000000000000007105 ) ) ;
#7434=ORIENTED_EDGE ( 'NONE', *, *, #3430, .F. ) ;
#7457=DIRECTION ( 'NONE',  ( 1.000000000000000000, 0.000000000000000000, 0.000000000000000000 ) ) ;
#7461=VECTOR ( 'NONE', #7805, 1000.000000000000000 ) ;
#7472=AXIS2_PLACEMENT_3D ( 'NONE', #7421, #8380, #1657 ) ;
#7490=DIRECTION ( 'NONE',  ( 0.000000000000000000, 0.000000000000000000, 1.000000000000000000 ) ) ;
#7525=ORIENTED_EDGE ( 'NONE', *, *, #9870, .T. ) ;
#7537=DIRECTION ( 'NONE',  ( 0.000000000000000000, 0.000000000000000000, 1.000000000000000000 ) ) ;
#7548=PLANE ( 'NONE',  #14031 ) ;
#7580=CARTESIAN_POINT ( 'NONE',  ( -18.12748877629581656, 43.82334295289051340, 0.000000000000000000 ) ) ;
#7602=DIRECTION ( 'NONE',  ( 0.000000000000000000, 0.000000000000000000, -1.000000000000000000 ) ) ;
#7614=DIRECTION ( 'NONE',  ( -4.625929269271486900E-16, 1.000000000000000000, 0.000000000000000000 ) ) ;
#7645=CARTESIAN_POINT ( 'NONE',  ( 18.12748877629582367, 43.82334295289049919, 0.000000000000000000 ) ) ;
#7647=AXIS2_PLACEMENT_3D ( 'NONE', #11945, #13201, #2218 ) ;
#7667=CARTESIAN_POINT ( 'NONE',  ( 0.000000000000000000, 25.49999999999996803, 8.000000000000007105 ) ) ;
#7676=ORIENTED_EDGE ( 'NONE', *, *, #11540, .T. ) ;
#7678=DIRECTION ( 'NONE',  ( 0.000000000000000000, 0.000000000000000000, 1.000000000000000000 ) ) ;
#7711=VECTOR ( 'NONE', #8020, 1000.000000000000000 ) ;
#7713=VECTOR ( 'NONE', #1635, 1000.000000000000114 ) ;
#7717=ORIENTED_EDGE ( 'NONE', *, *, #4834, .F. ) ;
#7721=LINE ( 'NONE', #6693, #6242 ) ;
#7726=CARTESIAN_POINT ( 'NONE',  ( 28.00000000000000355, 24.50000000000001421, 8.000000000000007105 ) ) ;
#7746=CARTESIAN_POINT ( 'NONE',  ( 3.822382184081044798, 10.25936179483148969, 8.000000000000007105 ) ) ;
#7763=ORIENTED_EDGE ( 'NONE', *, *, #8065, .T. ) ;
#7778=AXIS2_PLACEMENT_3D ( 'NONE', #13575, #7987, #12464 ) ;
#7779=ORIENTED_EDGE ( 'NONE', *, *, #5427, .T. ) ;
#7781=PLANE ( 'NONE',  #7778 ) ;
#7801=VECTOR ( 'NONE', #4537, 1000.000000000000000 ) ;
#7804=ORIENTED_EDGE ( 'NONE', *, *, #11283, .T. ) ;
#7805=DIRECTION ( 'NONE',  ( -0.9240638205168503205, 0.3822382184081049017, 0.000000000000000000 ) ) ;
#7808=CARTESIAN_POINT ( 'NONE',  ( 1.734723475976807094E-14, 35.49999999999996447, 0.000000000000000000 ) ) ;
#7821=CARTESIAN_POINT ( 'NONE',  ( -2.749999999999997780, 25.49999999999996803, 0.000000000000000000 ) ) ;
#7856=SHAPE_REPRESENTATION ( 'connector', ( #11025 ), #1463 ) ;
#7860=ORIENTED_EDGE ( 'NONE', *, *, #107, .T. ) ;
#7866=ADVANCED_FACE ( 'NONE', ( #817 ), #12158, .F. ) ;
#7867=ORIENTED_EDGE ( 'NONE', *, *, #620, .T. ) ;
#7875=CARTESIAN_POINT ( 'NONE',  ( 31.44014396567294867, 21.68342561534834090, 8.000000000000007105 ) ) ;
#7892=DIRECTION ( 'NONE',  ( 0.000000000000000000, 0.000000000000000000, -1.000000000000000000 ) ) ;
#7917=EDGE_CURVE ( 'NONE', #780, #8354, #10709, .T. ) ;
#7933=EDGE_CURVE ( 'NONE', #8755, #5025, #9539, .T. ) ;
#7945=DIRECTION ( 'NONE',  ( 0.000000000000000000, 0.000000000000000000, 1.000000000000000000 ) ) ;
#7958=ORIENTED_EDGE ( 'NONE', *, *, #8734, .T. ) ;
#7982=SURFACE_SIDE_STYLE ('',( #6312 ) ) ;
#7987=DIRECTION ( 'NONE',  ( -4.625929269271486900E-16, -1.000000000000000000, 0.000000000000000000 ) ) ;
#7991=CARTESIAN_POINT ( 'NONE',  ( 28.00000000000000355, 29.99999999999999645, 8.000000000000007105 ) ) ;
#8017=DIRECTION ( 'NONE',  ( 0.000000000000000000, 0.000000000000000000, -1.000000000000000000 ) ) ;
#8020=DIRECTION ( 'NONE',  ( 0.000000000000000000, 0.000000000000000000, -1.000000000000000000 ) ) ;
#8028=CARTESIAN_POINT ( 'NONE',  ( -2.749999999999997780, 25.49999999999996803, 8.000000000000007105 ) ) ;
#8030=EDGE_LOOP ( 'NONE', ( #4779, #4406, #1370, #2265 ) ) ;
#8048=VERTEX_POINT ( 'NONE', #5631 ) ;
#8065=EDGE_CURVE ( 'NONE', #8354, #10068, #1522, .T. ) ;
#8083=CARTESIAN_POINT ( 'NONE',  ( 28.00000000000000355, 35.49999999999997868, 8.000000000000007105 ) ) ;
#8084=DIRECTION ( 'NONE',  ( 1.000000000000000000, 4.625929269271485914E-16, 0.000000000000000000 ) ) ;
#8086=CARTESIAN_POINT ( 'NONE',  ( -2.750000000000003997, 40.49999999999999289, 0.000000000000000000 ) ) ;
#8095=LINE ( 'NONE', #2334, #7345 ) ;
#8121=EDGE_CURVE ( 'NONE', #6929, #7126, #2289, .T. ) ;
#8131=ORIENTED_EDGE ( 'NONE', *, *, #10025, .F. ) ;
#8133=DIRECTION ( 'NONE',  ( 1.000000000000000000, 0.000000000000000000, 0.000000000000000000 ) ) ;
#8135=DIRECTION ( 'NONE',  ( -1.000000000000000000, 0.000000000000000000, 0.000000000000000000 ) ) ;
#8143=ORIENTED_EDGE ( 'NONE', *, *, #12577, .F. ) ;
#8155=PLANE ( 'NONE',  #9816 ) ;
#8162=COLOUR_RGB ( '', 0.66274510, 0.83137255, 0.94901961) ;
#8171=ORIENTED_EDGE ( 'NONE', *, *, #381, .T. ) ;
#8182=CIRCLE ( 'NONE', #7472, 9.000000000000005329 ) ;
#8213=CARTESIAN_POINT ( 'NONE',  ( -6.938893903907228378E-15, 24.50000000000002132, 8.000000000000007105 ) ) ;
#8240=CARTESIAN_POINT ( 'NONE',  ( 13.00000000000000355, 24.50000000000001421, 8.000000000000007105 ) ) ;
#8275=ORIENTED_EDGE ( 'NONE', *, *, #11562, .F. ) ;
#8284=FACE_OUTER_BOUND ( 'NONE', #8798, .T. ) ;
#8285=FACE_OUTER_BOUND ( 'NONE', #11648, .T. ) ;
#8323=EDGE_CURVE ( 'NONE', #11470, #1840, #11160, .T. ) ;
#8324=CARTESIAN_POINT ( 'NONE',  ( -28.00000000000000355, 29.99999999999999645, 0.000000000000000000 ) ) ;
#8331=EDGE_CURVE ( 'NONE', #12327, #11314, #7721, .T. ) ;
#8332=ORIENTED_EDGE ( 'NONE', *, *, #12577, .T. ) ;
#8345=ADVANCED_FACE ( 'NONE', ( #13233 ), #1069, .F. ) ;
#8347=EDGE_CURVE ( 'NONE', #7126, #12483, #11150, .T. ) ;
#8354=VERTEX_POINT ( 'NONE', #12411 ) ;
#8365=DIRECTION ( 'NONE',  ( 0.000000000000000000, 0.000000000000000000, -1.000000000000000000 ) ) ;
#8370=AXIS2_PLACEMENT_3D ( 'NONE', #5894, #6732, #12307 ) ;
#8380=DIRECTION ( 'NONE',  ( 0.000000000000000000, 0.000000000000000000, 1.000000000000000000 ) ) ;
#8399=FACE_OUTER_BOUND ( 'NONE', #2835, .T. ) ;
#8407=ORIENTED_EDGE ( 'NONE', *, *, #4693, .T. ) ;
#8431=DIRECTION ( 'NONE',  ( 0.000000000000000000, 0.000000000000000000, -1.000000000000000000 ) ) ;
#8439=ORIENTED_EDGE ( 'NONE', *, *, #1500, .T. ) ;
#8471=ORIENTED_EDGE ( 'NONE', *, *, #8121, .F. ) ;
#8478=DIRECTION ( 'NONE',  ( -0.9240638205168504316, -0.3822382184081047352, 0.000000000000000000 ) ) ;
#8499=ORIENTED_EDGE ( 'NONE', *, *, #9960, .F. ) ;
#8507=EDGE_CURVE ( 'NONE', #11163, #11047, #10723, .T. ) ;
#8510=DIRECTION ( 'NONE',  ( 0.000000000000000000, 0.000000000000000000, -1.000000000000000000 ) ) ;
#8516=ORIENTED_EDGE ( 'NONE', *, *, #11605, .F. ) ;
#8539=DIRECTION ( 'NONE',  ( 1.000000000000000000, 0.000000000000000000, 0.000000000000000000 ) ) ;
#8558=DIRECTION ( 'NONE',  ( 0.000000000000000000, 0.000000000000000000, -1.000000000000000000 ) ) ;
#8563=VECTOR ( 'NONE', #8713, 1000.000000000000000 ) ;
#8601=EDGE_LOOP ( 'NONE', ( #10801, #13101, #1734, #5899 ) ) ;
#8630=CARTESIAN_POINT ( 'NONE',  ( 0.000000000000000000, 25.49999999999996803, 0.000000000000000000 ) ) ;
#8711=CARTESIAN_POINT ( 'NONE',  ( -13.00000000000000533, 35.49999999999997158, 8.000000000000007105 ) ) ;
#8713=DIRECTION ( 'NONE',  ( 0.000000000000000000, 0.000000000000000000, -1.000000000000000000 ) ) ;
#8734=EDGE_CURVE ( 'NONE', #11470, #36, #8812, .T. ) ;
#8737=VECTOR ( 'NONE', #2236, 1000.000000000000000 ) ;
#8755=VERTEX_POINT ( 'NONE', #8086 ) ;
#8786=DIRECTION ( 'NONE',  ( 0.000000000000000000, 0.000000000000000000, -1.000000000000000000 ) ) ;
#8798=EDGE_LOOP ( 'NONE', ( #683, #4156, #4389, #12824 ) ) ;
#8812=CIRCLE ( 'NONE', #2500, 9.999999999999996447 ) ;
#8823=ORIENTED_EDGE ( 'NONE', *, *, #3685, .T. ) ;
#8831=DIRECTION ( 'NONE',  ( 0.3822382184081047352, -0.9240638205168504316, -0.000000000000000000 ) ) ;
#8847=APPLICATION_CONTEXT ( 'automotive_design' ) ;
#8854=DIRECTION ( 'NONE',  ( -1.000000000000000000, 0.000000000000000000, 0.000000000000000000 ) ) ;
#8881=CIRCLE ( 'NONE', #11687, 5.499999999999976907 ) ;
#8889=EDGE_CURVE ( 'NONE', #10071, #9740, #13508, .T. ) ;
#8901=DIRECTION ( 'NONE',  ( 0.9240638205168504316, 0.3822382184081047352, 0.000000000000000000 ) ) ;
#8914=CIRCLE ( 'NONE', #246, 2.750000000000003997 ) ;
#8926=AXIS2_PLACEMENT_3D ( 'NONE', #9334, #9489, #12773 ) ;
#8951=CARTESIAN_POINT ( 'NONE',  ( 2.749999999999997780, 25.49999999999996803, 0.000000000000000000 ) ) ;
#8969=VERTEX_POINT ( 'NONE', #9872 ) ;
#8975=CARTESIAN_POINT ( 'NONE',  ( 2.749999999999997780, 25.49999999999996803, 8.000000000000007105 ) ) ;
#8985=EDGE_LOOP ( 'NONE', ( #8332, #4296, #5512, #11367, #8471 ) ) ;
#8987=CARTESIAN_POINT ( 'NONE',  ( 13.00000000000000533, 35.49999999999997158, 8.000000000000007105 ) ) ;
#9033=CARTESIAN_POINT ( 'NONE',  ( 18.12748877629582367, 43.82334295289049919, 8.000000000000007105 ) ) ;
#9041=VERTEX_POINT ( 'NONE', #13180 ) ;
#9042=DIRECTION ( 'NONE',  ( 1.000000000000000000, 0.000000000000000000, 0.000000000000000000 ) ) ;
#9050=ORIENTED_EDGE ( 'NONE', *, *, #6173, .T. ) ;
#9069=CIRCLE ( 'NONE', #9547, 10.00000000000000355 ) ;
#9089=DIRECTION ( 'NONE',  ( 0.000000000000000000, 0.000000000000000000, -1.000000000000000000 ) ) ;
#9130=CIRCLE ( 'NONE', #503, 2.750000000000003997 ) ;
#9157=DIRECTION ( 'NONE',  ( 0.000000000000000000, 0.000000000000000000, 1.000000000000000000 ) ) ;
#9165=FACE_OUTER_BOUND ( 'NONE', #1386, .T. ) ;
#9174=ORIENTED_EDGE ( 'NONE', *, *, #9224, .F. ) ;
#9197=AXIS2_PLACEMENT_3D ( 'NONE', #7991, #3557, #2442 ) ;
#9218=EDGE_CURVE ( 'NONE', #11189, #5462, #2400, .T. ) ;
#9222=DIRECTION ( 'NONE',  ( 0.000000000000000000, 0.000000000000000000, -1.000000000000000000 ) ) ;
#9224=EDGE_CURVE ( 'NONE', #10181, #12327, #1438, .T. ) ;
#9243=DIRECTION ( 'NONE',  ( 0.000000000000000000, 0.000000000000000000, 1.000000000000000000 ) ) ;
#9251=DIRECTION ( 'NONE',  ( 0.000000000000000000, 0.000000000000000000, -1.000000000000000000 ) ) ;
#9260=FACE_OUTER_BOUND ( 'NONE', #9651, .T. ) ;
#9276=EDGE_LOOP ( 'NONE', ( #9050, #13679, #10092, #11021, #7958, #10298, #3315, #7867, #2690 ) ) ;
#9290=CARTESIAN_POINT ( 'NONE',  ( 3.822382184081048351, 49.74063820516850143, 0.000000000000000000 ) ) ;
#9299=LINE ( 'NONE', #13780, #4708 ) ;
#9316=DIRECTION ( 'NONE',  ( -1.000000000000000000, 0.000000000000000000, 0.000000000000000000 ) ) ;
#9317=FACE_OUTER_BOUND ( 'NONE', #1674, .T. ) ;
#9325=FACE_OUTER_BOUND ( 'NONE', #4798, .T. ) ;
#9330=VERTEX_POINT ( 'NONE', #1744 ) ;
#9334=CARTESIAN_POINT ( 'NONE',  ( -28.00000000000000355, 29.99999999999999645, 0.000000000000000000 ) ) ;
#9340=CARTESIAN_POINT ( 'NONE',  ( 3.822382184081048351, 49.74063820516850143, 8.000000000000007105 ) ) ;
#9348=LINE ( 'NONE', #13834, #6853 ) ;
#9380=ORIENTED_EDGE ( 'NONE', *, *, #8331, .F. ) ;
#9392=CARTESIAN_POINT ( 'NONE',  ( 13.00000000000000533, 29.99999999999999289, 8.000000000000007105 ) ) ;
#9397=VECTOR ( 'NONE', #2011, 1000.000000000000000 ) ;
#9426=CIRCLE ( 'NONE', #7322, 9.000000000000001776 ) ;
#9453=ORIENTED_EDGE ( 'NONE', *, *, #13465, .F. ) ;
#9485=VECTOR ( 'NONE', #4771, 1000.000000000000000 ) ;
#9489=DIRECTION ( 'NONE',  ( 0.000000000000000000, 0.000000000000000000, 1.000000000000000000 ) ) ;
#9510=CARTESIAN_POINT ( 'NONE',  ( -33.49999999999998579, 29.99999999999999645, 8.000000000000007105 ) ) ;
#9516=FACE_OUTER_BOUND ( 'NONE', #3527, .T. ) ;
#9539=CIRCLE ( 'NONE', #7647, 2.750000000000003997 ) ;
#9547=AXIS2_PLACEMENT_3D ( 'NONE', #14182, #9848, #13018 ) ;
#9550=CYLINDRICAL_SURFACE ( 'NONE', #4927, 9.000000000000001776 ) ;
#9554=LINE ( 'NONE', #14237, #9397 ) ;
#9582=CARTESIAN_POINT ( 'NONE',  ( 0.000000000000000000, 19.49999999999999645, 8.000000000000007105 ) ) ;
#9607=CARTESIAN_POINT ( 'NONE',  ( -31.44014396567295577, 38.31657438465165200, 0.000000000000000000 ) ) ;
#9627=ORIENTED_EDGE ( 'NONE', *, *, #312, .T. ) ;
#9643=MECHANICAL_DESIGN_GEOMETRIC_PRESENTATION_REPRESENTATION('',(#3820),#6369);
#9651=EDGE_LOOP ( 'NONE', ( #7407, #8275, #10804, #4752 ) ) ;
#9689=ORIENTED_EDGE ( 'NONE', *, *, #7917, .F. ) ;
#9693=CARTESIAN_POINT ( 'NONE',  ( -13.00000000000000533, 24.50000000000001421, 8.000000000000007105 ) ) ;
#9696=VECTOR ( 'NONE', #4816, 1000.000000000000000 ) ;
#9721=DIRECTION ( 'NONE',  ( -1.000000000000000000, -2.312964634635743450E-16, 0.000000000000000000 ) ) ;
#9728=CARTESIAN_POINT ( 'NONE',  ( 31.44014396567294867, 21.68342561534834090, 0.000000000000000000 ) ) ;
#9730=ADVANCED_FACE ( 'NONE', ( #8285 ), #3851, .F. ) ;
#9732=ADVANCED_FACE ( 'NONE', ( #9317 ), #12681, .F. ) ;
#9738=LINE ( 'NONE', #5749, #11924 ) ;
#9740=VERTEX_POINT ( 'NONE', #7186 ) ;
#9747=DIRECTION ( 'NONE',  ( -1.000000000000000000, 0.000000000000000000, 0.000000000000000000 ) ) ;
#9751=( NAMED_UNIT ( * ) PLANE_ANGLE_UNIT ( ) SI_UNIT ( $, .RADIAN. ) );
#9793=PRODUCT_CONTEXT ( 'NONE', #3629, 'mechanical' ) ;
#9797=VERTEX_POINT ( 'NONE', #6009 ) ;
#9805=EDGE_CURVE ( 'NONE', #9041, #11047, #12810, .T. ) ;
#9816=AXIS2_PLACEMENT_3D ( 'NONE', #414, #4875, #13605 ) ;
#9826=CIRCLE ( 'NONE', #5153, 5.499999999999980460 ) ;
#9848=DIRECTION ( 'NONE',  ( 0.000000000000000000, 0.000000000000000000, 1.000000000000000000 ) ) ;
#9870=EDGE_CURVE ( 'NONE', #14193, #8048, #6348, .T. ) ;
#9872=CARTESIAN_POINT ( 'NONE',  ( -31.44014396567295577, 38.31657438465165200, 8.000000000000007105 ) ) ;
#9875=DIRECTION ( 'NONE',  ( 0.000000000000000000, 0.000000000000000000, 1.000000000000000000 ) ) ;
#9893=EDGE_CURVE ( 'NONE', #7396, #974, #3254, .T. ) ;
#9904=PRODUCT_DEFINITION_FORMATION_WITH_SPECIFIED_SOURCE ( 'ANY', '', #11629, .NOT_KNOWN. ) ;
#9922=DIRECTION ( 'NONE',  ( 0.000000000000000000, 0.000000000000000000, -1.000000000000000000 ) ) ;
#9935=DIRECTION ( 'NONE',  ( 0.000000000000000000, 0.000000000000000000, -1.000000000000000000 ) ) ;
#9939=ORIENTED_EDGE ( 'NONE', *, *, #2799, .F. ) ;
#9960=EDGE_CURVE ( 'NONE', #1865, #4996, #2971, .T. ) ;
#9997=DIRECTION ( 'NONE',  ( 1.000000000000000000, 0.000000000000000000, 0.000000000000000000 ) ) ;
#10012=ADVANCED_FACE ( 'NONE', ( #7405 ), #11963, .F. ) ;
#10020=FILL_AREA_STYLE ('',( #4414 ) ) ;
#10025=EDGE_CURVE ( 'NONE', #4996, #1788, #894, .T. ) ;
#10035=DIRECTION ( 'NONE',  ( 0.000000000000000000, 0.000000000000000000, 1.000000000000000000 ) ) ;
#10042=EDGE_CURVE ( 'NONE', #8048, #14193, #525, .T. ) ;
#10045=ORIENTED_EDGE ( 'NONE', *, *, #1919, .F. ) ;
#10064=CARTESIAN_POINT ( 'NONE',  ( 13.00000000000000533, 29.99999999999999289, 8.000000000000007105 ) ) ;
#10068=VERTEX_POINT ( 'NONE', #4508 ) ;
#10071=VERTEX_POINT ( 'NONE', #445 ) ;
#10092=ORIENTED_EDGE ( 'NONE', *, *, #2139, .T. ) ;
#10104=CARTESIAN_POINT ( 'NONE',  ( 6.938893903907228378E-15, 24.50000000000002132, 0.000000000000000000 ) ) ;
#10109=CIRCLE ( 'NONE', #11762, 2.749999999999997780 ) ;
#10111=DIRECTION ( 'NONE',  ( 1.000000000000000000, 0.000000000000000000, 0.000000000000000000 ) ) ;
#10114=DIRECTION ( 'NONE',  ( 0.000000000000000000, 0.000000000000000000, 1.000000000000000000 ) ) ;
#10144=ORIENTED_EDGE ( 'NONE', *, *, #10256, .F. ) ;
#10148=LINE ( 'NONE', #9033, #7801 ) ;
#10157=ADVANCED_FACE ( 'NONE', ( #10615, #7230, #600, #2945, #13038 ), #4120, .F. ) ;
#10179=PLANE ( 'NONE',  #3276 ) ;
#10181=VERTEX_POINT ( 'NONE', #4040 ) ;
#10204=ORIENTED_EDGE ( 'NONE', *, *, #6735, .T. ) ;
#10229=ORIENTED_EDGE ( 'NONE', *, *, #9805, .T. ) ;
#10256=EDGE_CURVE ( 'NONE', #974, #9330, #1440, .T. ) ;
#10262=DIRECTION ( 'NONE',  ( 0.000000000000000000, 0.000000000000000000, 1.000000000000000000 ) ) ;
#10276=CIRCLE ( 'NONE', #10532, 10.00000000000000355 ) ;
#10298=ORIENTED_EDGE ( 'NONE', *, *, #312, .F. ) ;
#10301=EDGE_CURVE ( 'NONE', #5025, #8755, #8914, .T. ) ;
#10329=VECTOR ( 'NONE', #3945, 1000.000000000000000 ) ;
#10384=DIRECTION ( 'NONE',  ( 1.000000000000000000, 0.000000000000000000, 0.000000000000000000 ) ) ;
#10410=AXIS2_PLACEMENT_3D ( 'NONE', #690, #8510, #9747 ) ;
#10414=CYLINDRICAL_SURFACE ( 'NONE', #2778, 5.499999999999975131 ) ;
#10421=CYLINDRICAL_SURFACE ( 'NONE', #10586, 2.749999999999997780 ) ;
#10461=ORIENTED_EDGE ( 'NONE', *, *, #9893, .T. ) ;
#10504=VERTEX_POINT ( 'NONE', #7136 ) ;
#10532=AXIS2_PLACEMENT_3D ( 'NONE', #13963, #717, #8539 ) ;
#10586=AXIS2_PLACEMENT_3D ( 'NONE', #13951, #9251, #405 ) ;
#10590=LINE ( 'NONE', #8083, #1607 ) ;
#10601=VERTEX_POINT ( 'NONE', #9340 ) ;
#10605=CARTESIAN_POINT ( 'NONE',  ( -3.822382184081048351, 49.74063820516850143, 8.000000000000007105 ) ) ;
#10615=FACE_BOUND ( 'NONE', #12138, .T. ) ;
#10618=DIRECTION ( 'NONE',  ( 0.000000000000000000, 0.000000000000000000, 1.000000000000000000 ) ) ;
#10641=CARTESIAN_POINT ( 'NONE',  ( -37.00000000000000711, 29.99999999999999645, 8.000000000000007105 ) ) ;
#10662=ADVANCED_FACE ( 'NONE', ( #4 ), #4275, .F. ) ;
#10687=EDGE_LOOP ( 'NONE', ( #5869, #6060, #14363, #7303 ) ) ;
#10709=CIRCLE ( 'NONE', #13996, 5.499999999999976907 ) ;
#10712=CARTESIAN_POINT ( 'NONE',  ( -18.12748877629581656, 43.82334295289051340, 8.000000000000007105 ) ) ;
#10723=LINE ( 'NONE', #3055, #3222 ) ;
#10740=AXIS2_PLACEMENT_3D ( 'NONE', #7225, #13979, #12876 ) ;
#10779=ORIENTED_EDGE ( 'NONE', *, *, #13068, .F. ) ;
#10799=AXIS2_PLACEMENT_3D ( 'NONE', #697, #7614, #5151 ) ;
#10801=ORIENTED_EDGE ( 'NONE', *, *, #13972, .T. ) ;
#10802=FACE_OUTER_BOUND ( 'NONE', #359, .T. ) ;
#10804=ORIENTED_EDGE ( 'NONE', *, *, #6173, .F. ) ;
#10838=( LENGTH_UNIT ( ) NAMED_UNIT ( * ) SI_UNIT ( .MILLI., .METRE. ) );
#10848=UNCERTAINTY_MEASURE_WITH_UNIT (LENGTH_MEASURE( 1.000000000000000082E-05 ), #11208, 'distance_accuracy_value', 'NONE');
#10854=DIRECTION ( 'NONE',  ( -1.000000000000000000, -2.312964634635743450E-16, 0.000000000000000000 ) ) ;
#10921=ORIENTED_EDGE ( 'NONE', *, *, #4220, .F. ) ;
#10952=ORIENTED_EDGE ( 'NONE', *, *, #107, .F. ) ;
#10991=ORIENTED_EDGE ( 'NONE', *, *, #8065, .F. ) ;
#11021=ORIENTED_EDGE ( 'NONE', *, *, #8323, .F. ) ;
#11025=AXIS2_PLACEMENT_3D ( 'NONE', #167, #6524, #5441 ) ;
#11031=CARTESIAN_POINT ( 'NONE',  ( -28.00000000000000355, 29.99999999999999645, 0.000000000000000000 ) ) ;
#11038=EDGE_LOOP ( 'NONE', ( #12544, #12699, #13787, #6866 ) ) ;
#11047=VERTEX_POINT ( 'NONE', #6877 ) ;
#11050=SURFACE_STYLE_FILL_AREA ( #10020 ) ;
#11076=ORIENTED_EDGE ( 'NONE', *, *, #9893, .F. ) ;
#11085=LINE ( 'NONE', #6684, #8737 ) ;
#11089=CARTESIAN_POINT ( 'NONE',  ( 13.00000000000000355, 24.50000000000001421, 8.000000000000007105 ) ) ;
#11107=DIRECTION ( 'NONE',  ( 1.000000000000000000, 0.000000000000000000, 0.000000000000000000 ) ) ;
#11132=ORIENTED_EDGE ( 'NONE', *, *, #5481, .F. ) ;
#11141=ORIENTED_EDGE ( 'NONE', *, *, #13972, .F. ) ;
#11150=CIRCLE ( 'NONE', #13500, 5.499999999999976907 ) ;
#11153=DIRECTION ( 'NONE',  ( 0.000000000000000000, 0.000000000000000000, -1.000000000000000000 ) ) ;
#11160=LINE ( 'NONE', #2249, #3681 ) ;
#11162=AXIS2_PLACEMENT_3D ( 'NONE', #12865, #12953, #14257 ) ;
#11163=VERTEX_POINT ( 'NONE', #2714 ) ;
#11189=VERTEX_POINT ( 'NONE', #1461 ) ;
#11208=( LENGTH_UNIT ( ) NAMED_UNIT ( * ) SI_UNIT ( .MILLI., .METRE. ) );
#11227=PLANE ( 'NONE',  #13766 ) ;
#11230=CARTESIAN_POINT ( 'NONE',  ( 7.500000000000029310, 29.99999999999999289, 8.000000000000007105 ) ) ;
#11283=EDGE_CURVE ( 'NONE', #904, #144, #507, .T. ) ;
#11285=DIRECTION ( 'NONE',  ( -1.000000000000000000, 0.000000000000000000, 0.000000000000000000 ) ) ;
#11306=VERTEX_POINT ( 'NONE', #13108 ) ;
#11314=VERTEX_POINT ( 'NONE', #13984 ) ;
#11367=ORIENTED_EDGE ( 'NONE', *, *, #8347, .F. ) ;
#11381=PRODUCT_DEFINITION_SHAPE ( 'NONE', 'NONE',  #4990 ) ;
#11393=ORIENTED_EDGE ( 'NONE', *, *, #4843, .F. ) ;
#11416=VECTOR ( 'NONE', #4725, 1000.000000000000000 ) ;
#11424=ORIENTED_EDGE ( 'NONE', *, *, #8331, .T. ) ;
#11469=LINE ( 'NONE', #8028, #9696 ) ;
#11470=VERTEX_POINT ( 'NONE', #1155 ) ;
#11475=DIRECTION ( 'NONE',  ( 0.000000000000000000, 0.000000000000000000, -1.000000000000000000 ) ) ;
#11489=LINE ( 'NONE', #13779, #9485 ) ;
#11524=DIRECTION ( 'NONE',  ( 0.000000000000000000, 0.000000000000000000, 1.000000000000000000 ) ) ;
#11540=EDGE_CURVE ( 'NONE', #4996, #6397, #9826, .T. ) ;
#11562=EDGE_CURVE ( 'NONE', #8969, #3225, #5888, .T. ) ;
#11572=ORIENTED_EDGE ( 'NONE', *, *, #7237, .T. ) ;
#11586=ORIENTED_EDGE ( 'NONE', *, *, #2139, .F. ) ;
#11605=EDGE_CURVE ( 'NONE', #10601, #5280, #10276, .T. ) ;
#11609=DIRECTION ( 'NONE',  ( 0.000000000000000000, 0.000000000000000000, 1.000000000000000000 ) ) ;
#11629=PRODUCT ( 'connector', 'connector', '', ( #9793 ) ) ;
#11643=VECTOR ( 'NONE', #4743, 1000.000000000000000 ) ;
#11648=EDGE_LOOP ( 'NONE', ( #791, #4692, #781, #10461 ) ) ;
#11666=AXIS2_PLACEMENT_3D ( 'NONE', #11031, #7945, #1151 ) ;
#11687=AXIS2_PLACEMENT_3D ( 'NONE', #1808, #5308, #4233 ) ;
#11708=AXIS2_PLACEMENT_3D ( 'NONE', #3063, #7490, #13911 ) ;
#11712=VECTOR ( 'NONE', #1279, 1000.000000000000000 ) ;
#11750=VERTEX_POINT ( 'NONE', #13726 ) ;
#11762=AXIS2_PLACEMENT_3D ( 'NONE', #8630, #10618, #3160 ) ;
#11798=CLOSED_SHELL ( 'NONE', ( #13594, #1629, #2876, #12309, #3171, #5347, #10157, #5803, #11863, #12955, #6544, #6727, #1020, #6414, #912, #2956, #9730, #7866, #13894, #10012, #9732, #2721, #8345, #3879, #10662 ) ) ;
#11847=EDGE_CURVE ( 'NONE', #7126, #780, #12685, .T. ) ;
#11863=ADVANCED_FACE ( 'NONE', ( #13513 ), #9550, .T. ) ;
#11877=AXIS2_PLACEMENT_3D ( 'NONE', #3693, #10262, #8133 ) ;
#11888=VECTOR ( 'NONE', #8084, 1000.000000000000000 ) ;
#11904=VERTEX_POINT ( 'NONE', #699 ) ;
#11924=VECTOR ( 'NONE', #11475, 1000.000000000000000 ) ;
#11928=CARTESIAN_POINT ( 'NONE',  ( 0.000000000000000000, 40.49999999999999289, 8.000000000000007105 ) ) ;
#11945=CARTESIAN_POINT ( 'NONE',  ( 0.000000000000000000, 40.49999999999999289, 0.000000000000000000 ) ) ;
#11963=PLANE ( 'NONE',  #10799 ) ;
#11996=ORIENTED_EDGE ( 'NONE', *, *, #109, .F. ) ;
#12121=CARTESIAN_POINT ( 'NONE',  ( 28.00000000000000355, 29.99999999999999645, 8.000000000000007105 ) ) ;
#12138=EDGE_LOOP ( 'NONE', ( #3994, #2905, #2462, #5152, #7763 ) ) ;
#12145=CIRCLE ( 'NONE', #10740, 9.000000000000005329 ) ;
#12158=CYLINDRICAL_SURFACE ( 'NONE', #3024, 5.499999999999976907 ) ;
#12219=VECTOR ( 'NONE', #7602, 1000.000000000000000 ) ;
#12223=VERTEX_POINT ( 'NONE', #9290 ) ;
#12260=FACE_OUTER_BOUND ( 'NONE', #8601, .T. ) ;
#12275=ORIENTED_EDGE ( 'NONE', *, *, #6735, .F. ) ;
#12307=DIRECTION ( 'NONE',  ( 1.000000000000000000, 0.000000000000000000, 0.000000000000000000 ) ) ;
#12309=ADVANCED_FACE ( 'NONE', ( #9516 ), #2042, .F. ) ;
#12322=ORIENTED_EDGE ( 'NONE', *, *, #8507, .T. ) ;
#12327=VERTEX_POINT ( 'NONE', #9728 ) ;
#12334=LINE ( 'NONE', #11089, #2062 ) ;
#12381=ORIENTED_EDGE ( 'NONE', *, *, #6631, .T. ) ;
#12386=MECHANICAL_DESIGN_GEOMETRIC_PRESENTATION_REPRESENTATION('',(#1384),#2566);
#12411=CARTESIAN_POINT ( 'NONE',  ( 13.00000000000000355, 24.50000000000001421, 0.000000000000000000 ) ) ;
#12427=DIRECTION ( 'NONE',  ( 0.000000000000000000, 0.000000000000000000, 1.000000000000000000 ) ) ;
#12464=DIRECTION ( 'NONE',  ( 1.000000000000000000, -4.625929269271486900E-16, -0.000000000000000000 ) ) ;
#12483=VERTEX_POINT ( 'NONE', #8240 ) ;
#12494=CARTESIAN_POINT ( 'NONE',  ( -28.00000000000000355, 29.99999999999999645, 8.000000000000007105 ) ) ;
#12505=FACE_BOUND ( 'NONE', #8985, .T. ) ;
#12544=ORIENTED_EDGE ( 'NONE', *, *, #3685, .F. ) ;
#12577=EDGE_CURVE ( 'NONE', #6929, #9740, #2474, .T. ) ;
#12588=ORIENTED_EDGE ( 'NONE', *, *, #11540, .F. ) ;
#12593=VECTOR ( 'NONE', #6556, 1000.000000000000000 ) ;
#12594=UNCERTAINTY_MEASURE_WITH_UNIT (LENGTH_MEASURE( 1.000000000000000082E-05 ), #1937, 'distance_accuracy_value', 'NONE');
#12602=DIRECTION ( 'NONE',  ( 0.000000000000000000, 0.000000000000000000, -1.000000000000000000 ) ) ;
#12639=FACE_BOUND ( 'NONE', #3571, .T. ) ;
#12655=EDGE_LOOP ( 'NONE', ( #7779, #291, #12588, #8499, #14086 ) ) ;
#12659=CYLINDRICAL_SURFACE ( 'NONE', #12894, 2.750000000000003997 ) ;
#12668=COLOUR_RGB ( '', 0.66274510, 0.83137255, 0.94901961) ;
#12681=CYLINDRICAL_SURFACE ( 'NONE', #6019, 5.499999999999975131 ) ;
#12685=LINE ( 'NONE', #11230, #11712 ) ;
#12686=ORIENTED_EDGE ( 'NONE', *, *, #109, .T. ) ;
#12687=LINE ( 'NONE', #7115, #11416 ) ;
#12693=EDGE_LOOP ( 'NONE', ( #12275, #551, #2921, #845 ) ) ;
#12699=ORIENTED_EDGE ( 'NONE', *, *, #5105, .T. ) ;
#12758=DIRECTION ( 'NONE',  ( 2.312964634635743943E-16, -1.000000000000000000, -0.000000000000000000 ) ) ;
#12773=DIRECTION ( 'NONE',  ( 1.000000000000000000, 0.000000000000000000, 0.000000000000000000 ) ) ;
#12777=CARTESIAN_POINT ( 'NONE',  ( -37.00000000000000711, 29.99999999999999645, 8.000000000000007105 ) ) ;
#12793=DIRECTION ( 'NONE',  ( 0.000000000000000000, 0.000000000000000000, 1.000000000000000000 ) ) ;
#12810=CIRCLE ( 'NONE', #6484, 9.000000000000005329 ) ;
#12824=ORIENTED_EDGE ( 'NONE', *, *, #14458, .F. ) ;
#12834=ORIENTED_EDGE ( 'NONE', *, *, #8507, .F. ) ;
#12865=CARTESIAN_POINT ( 'NONE',  ( 28.00000000000000355, 29.99999999999999645, 8.000000000000007105 ) ) ;
#12869=ORIENTED_EDGE ( 'NONE', *, *, #4843, .T. ) ;
#12876=DIRECTION ( 'NONE',  ( 1.000000000000000000, 0.000000000000000000, 0.000000000000000000 ) ) ;
#12894=AXIS2_PLACEMENT_3D ( 'NONE', #4772, #9222, #11285 ) ;
#12898=CARTESIAN_POINT ( 'NONE',  ( -28.00000000000000355, 35.49999999999997868, 0.000000000000000000 ) ) ;
#12906=EDGE_LOOP ( 'NONE', ( #11132, #2138, #5293, #11141, #11424, #10779, #12322, #13057, #7434 ) ) ;
#12916=CYLINDRICAL_SURFACE ( 'NONE', #10410, 2.750000000000003997 ) ;
#12951=EDGE_LOOP ( 'NONE', ( #3880, #4800, #3861, #4791 ) ) ;
#12953=DIRECTION ( 'NONE',  ( 0.000000000000000000, 0.000000000000000000, 1.000000000000000000 ) ) ;
#12955=ADVANCED_FACE ( 'NONE', ( #14083 ), #14010, .T. ) ;
#13018=DIRECTION ( 'NONE',  ( 1.000000000000000000, 0.000000000000000000, 0.000000000000000000 ) ) ;
#13028=ORIENTED_EDGE ( 'NONE', *, *, #1593, .F. ) ;
#13038=FACE_BOUND ( 'NONE', #3296, .T. ) ;
#13039=DIRECTION ( 'NONE',  ( -1.000000000000000000, 0.000000000000000000, 0.000000000000000000 ) ) ;
#13057=ORIENTED_EDGE ( 'NONE', *, *, #9805, .F. ) ;
#13068=EDGE_CURVE ( 'NONE', #11163, #11314, #4738, .T. ) ;
#13070=DIRECTION ( 'NONE',  ( 0.000000000000000000, 0.000000000000000000, -1.000000000000000000 ) ) ;
#13091=EDGE_CURVE ( 'NONE', #9797, #11904, #3322, .T. ) ;
#13097=ORIENTED_EDGE ( 'NONE', *, *, #6631, .F. ) ;
#13101=ORIENTED_EDGE ( 'NONE', *, *, #4693, .F. ) ;
#13108=CARTESIAN_POINT ( 'NONE',  ( 31.44014396567294867, 38.31657438465161647, 8.000000000000007105 ) ) ;
#13112=ADVANCED_BREP_SHAPE_REPRESENTATION ( '', ( #1904, #11025 ), #1463 ) ;
#13180=CARTESIAN_POINT ( 'NONE',  ( -37.00000000000000711, 29.99999999999999645, 0.000000000000000000 ) ) ;
#13187=VECTOR ( 'NONE', #6552, 1000.000000000000000 ) ;
#13201=DIRECTION ( 'NONE',  ( 0.000000000000000000, 0.000000000000000000, 1.000000000000000000 ) ) ;
#13233=FACE_OUTER_BOUND ( 'NONE', #12951, .T. ) ;
#13349=PRODUCT_DEFINITION_CONTEXT ( 'detailed design', #8847, 'design' ) ;
#13354=SHAPE_REPRESENTATION_RELATIONSHIP ( 'NONE' , 'NONE' ,  #7856, #13112 ) ;
#13365=CARTESIAN_POINT ( 'NONE',  ( 0.000000000000000000, 19.49999999999999645, 8.000000000000007105 ) ) ;
#13393=AXIS2_PLACEMENT_3D ( 'NONE', #6588, #7678, #13487 ) ;
#13465=EDGE_CURVE ( 'NONE', #4572, #937, #10109, .T. ) ;
#13487=DIRECTION ( 'NONE',  ( 1.000000000000000000, 0.000000000000000000, 0.000000000000000000 ) ) ;
#13500=AXIS2_PLACEMENT_3D ( 'NONE', #10064, #6545, #9997 ) ;
#13508=CIRCLE ( 'NONE', #11162, 5.499999999999984013 ) ;
#13513=FACE_OUTER_BOUND ( 'NONE', #8030, .T. ) ;
#13530=CARTESIAN_POINT ( 'NONE',  ( -3.065261730689029740, 7.410293710401353984, 8.000000000000007105 ) ) ;
#13575=CARTESIAN_POINT ( 'NONE',  ( 1.734723475976807094E-14, 35.49999999999996447, 8.000000000000007105 ) ) ;
#13594=ADVANCED_FACE ( 'NONE', ( #9325 ), #10421, .F. ) ;
#13605=DIRECTION ( 'NONE',  ( 0.9240638205168504316, 0.3822382184081046796, 0.000000000000000000 ) ) ;
#13617=AXIS2_PLACEMENT_3D ( 'NONE', #5024, #413, #4947 ) ;
#13621=VECTOR ( 'NONE', #14305, 1000.000000000000000 ) ;
#13653=DIRECTION ( 'NONE',  ( 1.000000000000000000, 0.000000000000000000, 0.000000000000000000 ) ) ;
#13679=ORIENTED_EDGE ( 'NONE', *, *, #5896, .T. ) ;
#13685=CARTESIAN_POINT ( 'NONE',  ( -31.44014396567295577, 38.31657438465165200, 8.000000000000007105 ) ) ;
#13724=CARTESIAN_POINT ( 'NONE',  ( 0.000000000000000000, 25.49999999999996803, 8.000000000000007105 ) ) ;
#13726=CARTESIAN_POINT ( 'NONE',  ( -3.822382184081048351, 49.74063820516850143, 0.000000000000000000 ) ) ;
#13766=AXIS2_PLACEMENT_3D ( 'NONE', #1339, #5716, #3488 ) ;
#13779=CARTESIAN_POINT ( 'NONE',  ( 3.822382184081048351, 49.74063820516850143, 8.000000000000007105 ) ) ;
#13780=CARTESIAN_POINT ( 'NONE',  ( -3.822382184081048351, 49.74063820516850143, 8.000000000000007105 ) ) ;
#13787=ORIENTED_EDGE ( 'NONE', *, *, #13091, .T. ) ;
#13804=VECTOR ( 'NONE', #9935, 1000.000000000000000 ) ;
#13834=CARTESIAN_POINT ( 'NONE',  ( -3.065261730689029740, 7.410293710401353984, 8.000000000000007105 ) ) ;
#13835=EDGE_LOOP ( 'NONE', ( #7804, #12686, #3480, #11393 ) ) ;
#13839=CARTESIAN_POINT ( 'NONE',  ( 31.44014396567294867, 38.31657438465161647, 8.000000000000007105 ) ) ;
#13887=DIRECTION ( 'NONE',  ( 1.000000000000000000, 0.000000000000000000, 0.000000000000000000 ) ) ;
#13889=EDGE_LOOP ( 'NONE', ( #3785, #4188, #8143, #5071 ) ) ;
#13893=AXIS2_PLACEMENT_3D ( 'NONE', #14178, #1951, #6399 ) ;
#13894=ADVANCED_FACE ( 'NONE', ( #4641 ), #7781, .T. ) ;
#13896=LINE ( 'NONE', #12777, #7211 ) ;
#13911=DIRECTION ( 'NONE',  ( 1.000000000000000000, 0.000000000000000000, 0.000000000000000000 ) ) ;
#13951=CARTESIAN_POINT ( 'NONE',  ( 0.000000000000000000, 25.49999999999996803, 8.000000000000007105 ) ) ;
#13955=EDGE_LOOP ( 'NONE', ( #11586, #320, #10229, #10045 ) ) ;
#13963=CARTESIAN_POINT ( 'NONE',  ( 0.000000000000000000, 40.49999999999999289, 8.000000000000007105 ) ) ;
#13972=EDGE_CURVE ( 'NONE', #12327, #2267, #9426, .T. ) ;
#13979=DIRECTION ( 'NONE',  ( 0.000000000000000000, 0.000000000000000000, 1.000000000000000000 ) ) ;
#13984=CARTESIAN_POINT ( 'NONE',  ( 3.822382184081044798, 10.25936179483148969, 0.000000000000000000 ) ) ;
#13996=AXIS2_PLACEMENT_3D ( 'NONE', #3035, #7537, #7457 ) ;
#14010=PLANE ( 'NONE',  #3103 ) ;
#14019=LINE ( 'NONE', #10712, #7713 ) ;
#14023=CYLINDRICAL_SURFACE ( 'NONE', #2038, 5.499999999999984013 ) ;
#14031=AXIS2_PLACEMENT_3D ( 'NONE', #13530, #8831, #8901 ) ;
#14083=FACE_OUTER_BOUND ( 'NONE', #1537, .T. ) ;
#14086=ORIENTED_EDGE ( 'NONE', *, *, #3468, .F. ) ;
#14094=ORIENTED_EDGE ( 'NONE', *, *, #4834, .T. ) ;
#14152=CARTESIAN_POINT ( 'NONE',  ( 3.065261730689029740, 7.410293710401357536, 8.000000000000007105 ) ) ;
#14166=CARTESIAN_POINT ( 'NONE',  ( -28.00000000000000355, 29.99999999999999645, 8.000000000000007105 ) ) ;
#14178=CARTESIAN_POINT ( 'NONE',  ( 0.000000000000000000, 40.49999999999999289, 8.000000000000007105 ) ) ;
#14182=CARTESIAN_POINT ( 'NONE',  ( 0.000000000000000000, 40.49999999999999289, 0.000000000000000000 ) ) ;
#14193=VERTEX_POINT ( 'NONE', #6589 ) ;
#14234=DIRECTION ( 'NONE',  ( -1.000000000000000000, 4.625929269271485914E-16, 0.000000000000000000 ) ) ;
#14237=CARTESIAN_POINT ( 'NONE',  ( 13.00000000000000533, 35.49999999999997158, 8.000000000000007105 ) ) ;
#14257=DIRECTION ( 'NONE',  ( 1.000000000000000000, 0.000000000000000000, 0.000000000000000000 ) ) ;
#14269=DIRECTION ( 'NONE',  ( 1.000000000000000000, 0.000000000000000000, 0.000000000000000000 ) ) ;
#14283=CARTESIAN_POINT ( 'NONE',  ( -31.44014396567295577, 21.68342561534834445, 8.000000000000007105 ) ) ;
#14305=DIRECTION ( 'NONE',  ( 0.000000000000000000, 0.000000000000000000, -1.000000000000000000 ) ) ;
#14354=ORIENTED_EDGE ( 'NONE', *, *, #10042, .F. ) ;
#14357=( NAMED_UNIT ( * ) SI_UNIT ( $, .STERADIAN. ) SOLID_ANGLE_UNIT ( ) );
#14363=ORIENTED_EDGE ( 'NONE', *, *, #8734, .F. ) ;
#14409=CARTESIAN_POINT ( 'NONE',  ( 31.44014396567294867, 38.31657438465161647, 0.000000000000000000 ) ) ;
#14427=DIRECTION ( 'NONE',  ( -1.000000000000000000, 0.000000000000000000, 0.000000000000000000 ) ) ;
#14439=AXIS2_PLACEMENT_3D ( 'NONE', #12121, #2101, #1144 ) ;
#14442=CARTESIAN_POINT ( 'NONE',  ( -28.00000000000000355, 29.99999999999999645, 0.000000000000000000 ) ) ;
#14458=EDGE_CURVE ( 'NONE', #6929, #11189, #9554, .T. ) ;
ENDSEC;
END-ISO-10303-21;
